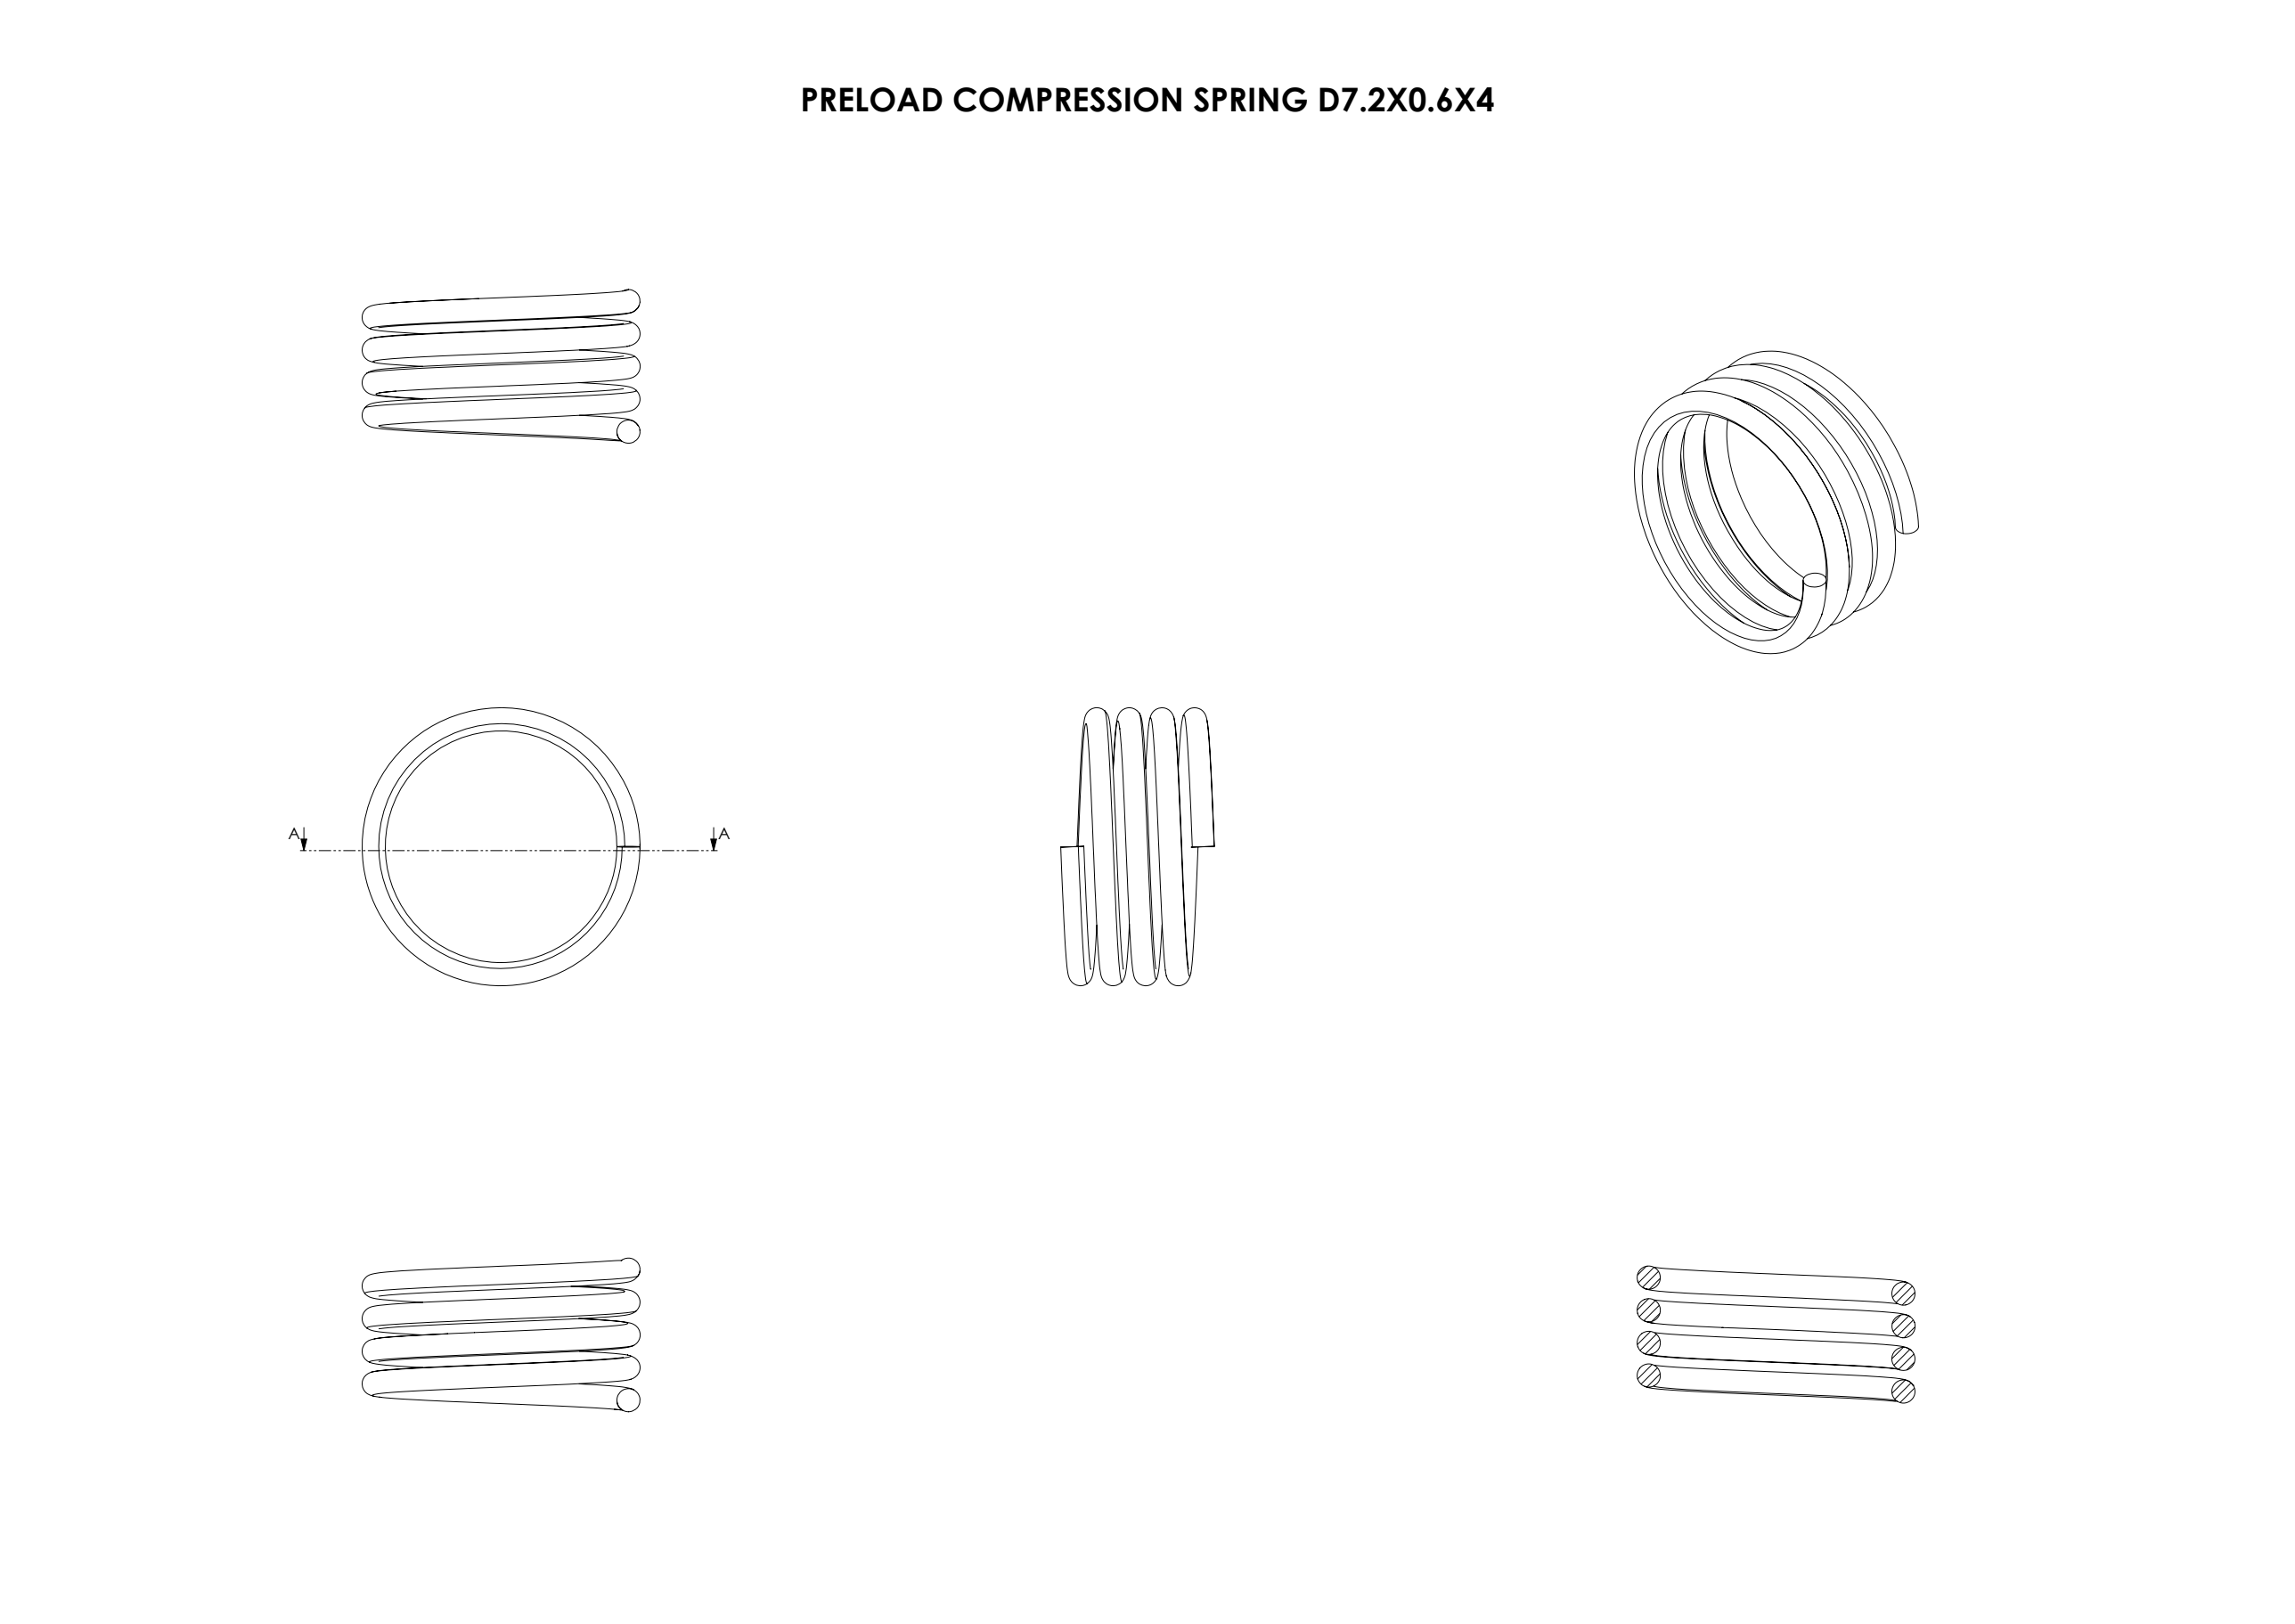
ISO-10303-21;
HEADER;
/* Generated by software containing ST-Developer
 * from STEP Tools, Inc. (www.steptools.com) 
 */

FILE_DESCRIPTION(
/* description */ (''),
/* implementation_level */ '2;1');

FILE_NAME(
/* name */ 
'10_Preload_Compression_Spring_D7.2x0.6x4.step',
/* time_stamp */ '2026-10-20T10:06:23-07:00',
/* author */ (''),
/* organization */ (''),
/* preprocessor_version */ 'ST-DEVELOPER v20.2',
/* originating_system */ 'Autodesk Translation Framework v15.15.0.0',
/* authorisation */ '');

FILE_SCHEMA (('AUTOMOTIVE_DESIGN { 1 0 10303 214 3 1 1 }'));
ENDSEC;

DATA;
#10=MECHANICAL_DESIGN_GEOMETRIC_PRESENTATION_REPRESENTATION('',(#471),#38611);
#443=SHAPE_REPRESENTATION_RELATIONSHIP('SRR','None',#38679,#457);
#457=ADVANCED_BREP_SHAPE_REPRESENTATION('',(#485),#38608);
#471=STYLED_ITEM('',(#38878),#485);
#485=MANIFOLD_SOLID_BREP('Spring',#16245);
#505=B_SPLINE_SURFACE_WITH_KNOTS('',3,3,((#31614,#31615,#31616,#31617,#31618,
#31619,#31620,#31621,#31622,#31623,#31624,#31625,#31626,#31627,#31628,#31629,
#31630,#31631,#31632,#31633,#31634,#31635,#31636,#31637,#31638,#31639,#31640,
#31641,#31642,#31643,#31644,#31645,#31646,#31647,#31648,#31649,#31650,#31651,
#31652,#31653,#31654,#31655,#31656,#31657,#31658,#31659,#31660,#31661,#31662,
#31663,#31664,#31665,#31666,#31667),(#31668,#31669,#31670,#31671,#31672,
#31673,#31674,#31675,#31676,#31677,#31678,#31679,#31680,#31681,#31682,#31683,
#31684,#31685,#31686,#31687,#31688,#31689,#31690,#31691,#31692,#31693,#31694,
#31695,#31696,#31697,#31698,#31699,#31700,#31701,#31702,#31703,#31704,#31705,
#31706,#31707,#31708,#31709,#31710,#31711,#31712,#31713,#31714,#31715,#31716,
#31717,#31718,#31719,#31720,#31721),(#31722,#31723,#31724,#31725,#31726,
#31727,#31728,#31729,#31730,#31731,#31732,#31733,#31734,#31735,#31736,#31737,
#31738,#31739,#31740,#31741,#31742,#31743,#31744,#31745,#31746,#31747,#31748,
#31749,#31750,#31751,#31752,#31753,#31754,#31755,#31756,#31757,#31758,#31759,
#31760,#31761,#31762,#31763,#31764,#31765,#31766,#31767,#31768,#31769,#31770,
#31771,#31772,#31773,#31774,#31775),(#31776,#31777,#31778,#31779,#31780,
#31781,#31782,#31783,#31784,#31785,#31786,#31787,#31788,#31789,#31790,#31791,
#31792,#31793,#31794,#31795,#31796,#31797,#31798,#31799,#31800,#31801,#31802,
#31803,#31804,#31805,#31806,#31807,#31808,#31809,#31810,#31811,#31812,#31813,
#31814,#31815,#31816,#31817,#31818,#31819,#31820,#31821,#31822,#31823,#31824,
#31825,#31826,#31827,#31828,#31829),(#31830,#31831,#31832,#31833,#31834,
#31835,#31836,#31837,#31838,#31839,#31840,#31841,#31842,#31843,#31844,#31845,
#31846,#31847,#31848,#31849,#31850,#31851,#31852,#31853,#31854,#31855,#31856,
#31857,#31858,#31859,#31860,#31861,#31862,#31863,#31864,#31865,#31866,#31867,
#31868,#31869,#31870,#31871,#31872,#31873,#31874,#31875,#31876,#31877,#31878,
#31879,#31880,#31881,#31882,#31883),(#31884,#31885,#31886,#31887,#31888,
#31889,#31890,#31891,#31892,#31893,#31894,#31895,#31896,#31897,#31898,#31899,
#31900,#31901,#31902,#31903,#31904,#31905,#31906,#31907,#31908,#31909,#31910,
#31911,#31912,#31913,#31914,#31915,#31916,#31917,#31918,#31919,#31920,#31921,
#31922,#31923,#31924,#31925,#31926,#31927,#31928,#31929,#31930,#31931,#31932,
#31933,#31934,#31935,#31936,#31937),(#31938,#31939,#31940,#31941,#31942,
#31943,#31944,#31945,#31946,#31947,#31948,#31949,#31950,#31951,#31952,#31953,
#31954,#31955,#31956,#31957,#31958,#31959,#31960,#31961,#31962,#31963,#31964,
#31965,#31966,#31967,#31968,#31969,#31970,#31971,#31972,#31973,#31974,#31975,
#31976,#31977,#31978,#31979,#31980,#31981,#31982,#31983,#31984,#31985,#31986,
#31987,#31988,#31989,#31990,#31991),(#31992,#31993,#31994,#31995,#31996,
#31997,#31998,#31999,#32000,#32001,#32002,#32003,#32004,#32005,#32006,#32007,
#32008,#32009,#32010,#32011,#32012,#32013,#32014,#32015,#32016,#32017,#32018,
#32019,#32020,#32021,#32022,#32023,#32024,#32025,#32026,#32027,#32028,#32029,
#32030,#32031,#32032,#32033,#32034,#32035,#32036,#32037,#32038,#32039,#32040,
#32041,#32042,#32043,#32044,#32045),(#32046,#32047,#32048,#32049,#32050,
#32051,#32052,#32053,#32054,#32055,#32056,#32057,#32058,#32059,#32060,#32061,
#32062,#32063,#32064,#32065,#32066,#32067,#32068,#32069,#32070,#32071,#32072,
#32073,#32074,#32075,#32076,#32077,#32078,#32079,#32080,#32081,#32082,#32083,
#32084,#32085,#32086,#32087,#32088,#32089,#32090,#32091,#32092,#32093,#32094,
#32095,#32096,#32097,#32098,#32099),(#32100,#32101,#32102,#32103,#32104,
#32105,#32106,#32107,#32108,#32109,#32110,#32111,#32112,#32113,#32114,#32115,
#32116,#32117,#32118,#32119,#32120,#32121,#32122,#32123,#32124,#32125,#32126,
#32127,#32128,#32129,#32130,#32131,#32132,#32133,#32134,#32135,#32136,#32137,
#32138,#32139,#32140,#32141,#32142,#32143,#32144,#32145,#32146,#32147,#32148,
#32149,#32150,#32151,#32152,#32153),(#32154,#32155,#32156,#32157,#32158,
#32159,#32160,#32161,#32162,#32163,#32164,#32165,#32166,#32167,#32168,#32169,
#32170,#32171,#32172,#32173,#32174,#32175,#32176,#32177,#32178,#32179,#32180,
#32181,#32182,#32183,#32184,#32185,#32186,#32187,#32188,#32189,#32190,#32191,
#32192,#32193,#32194,#32195,#32196,#32197,#32198,#32199,#32200,#32201,#32202,
#32203,#32204,#32205,#32206,#32207)),.UNSPECIFIED.,.T.,.F.,.F.,(4,1,1,1,
1,1,1,1,4),(4,1,1,1,1,1,1,1,1,1,1,1,1,1,1,1,1,1,1,1,1,1,1,1,1,1,1,1,1,1,
1,1,1,1,1,1,1,1,1,1,1,1,1,1,1,1,1,1,1,1,1,4),(-3.14159265358979,-2.46839422782055,
-2.24399475256414,-1.34639685153848,-0.448798950512828,0.448798950512828,
1.34639685153848,2.24399475256414,3.14159265358979),(0.,0.0178571428571429,
0.0357142857142857,0.0535714285714286,0.0714285714285714,0.0892857142857143,
0.107142857142857,0.125,0.133928571428571,0.138392857142857,0.142857142857143,
0.166666666666667,0.19047619047619,0.214285714285714,0.232142857142857,
0.25,0.267857142857143,0.285714285714286,0.303571428571429,0.321428571428571,
0.339285714285714,0.357142857142857,0.375,0.392857142857143,0.428571428571429,
0.464285714285714,0.5,0.535714285714286,0.553571428571429,0.571428571428571,
0.589285714285714,0.607142857142857,0.625,0.642857142857143,0.660714285714286,
0.678571428571428,0.696428571428571,0.714285714285714,0.738095238095238,
0.761904761904762,0.785714285714286,0.809523809523809,0.833333333333333,
0.857142857142857,0.875,0.892857142857143,0.910714285714286,0.928571428571429,
0.946428571428571,0.964285714285714,0.982142857142857,1.),.UNSPECIFIED.);
#728=B_SPLINE_CURVE_WITH_KNOTS('',3,(#32211,#32212,#32213,#32214,#32215,
#32216,#32217,#32218,#32219,#32220,#32221,#32222,#32223,#32224,#32225,#32226,
#32227,#32228,#32229,#32230,#32231,#32232,#32233,#32234,#32235,#32236,#32237,
#32238,#32239,#32240,#32241,#32242,#32243,#32244,#32245,#32246,#32247,#32248,
#32249,#32250,#32251,#32252,#32253,#32254,#32255,#32256,#32257,#32258,#32259,
#32260,#32261,#32262,#32263,#32264),.UNSPECIFIED.,.F.,.F.,(4,1,1,1,1,1,
1,1,1,1,1,1,1,1,1,1,1,1,1,1,1,1,1,1,1,1,1,1,1,1,1,1,1,1,1,1,1,1,1,1,1,1,
1,1,1,1,1,1,1,1,1,4),(0.,0.0178571428571429,0.0357142857142857,0.0535714285714286,
0.0714285714285714,0.0892857142857143,0.107142857142857,0.125,0.133928571428571,
0.138392857142857,0.142857142857143,0.166666666666667,0.19047619047619,
0.214285714285714,0.232142857142857,0.25,0.267857142857143,0.285714285714286,
0.303571428571429,0.321428571428571,0.339285714285714,0.357142857142857,
0.375,0.392857142857143,0.428571428571429,0.464285714285714,0.5,0.535714285714286,
0.553571428571429,0.571428571428571,0.589285714285714,0.607142857142857,
0.625,0.642857142857143,0.660714285714286,0.678571428571428,0.696428571428571,
0.714285714285714,0.738095238095238,0.761904761904762,0.785714285714286,
0.809523809523809,0.833333333333333,0.857142857142857,0.875,0.892857142857143,
0.910714285714286,0.928571428571429,0.946428571428571,0.964285714285714,
0.982142857142857,1.),.UNSPECIFIED.);
#1516=CIRCLE('',#17328,0.03);
#1517=CIRCLE('',#17329,0.03);
#2388=FACE_OUTER_BOUND('',#3348,.T.);
#2389=FACE_OUTER_BOUND('',#3349,.T.);
#2390=FACE_OUTER_BOUND('',#3350,.T.);
#3348=EDGE_LOOP('',(#13117,#13118,#13119,#13120));
#3349=EDGE_LOOP('',(#13121));
#3350=EDGE_LOOP('',(#13122));
#7074=VERTEX_POINT('',#32208);
#7075=VERTEX_POINT('',#32210);
#9174=EDGE_CURVE('',#7074,#7074,#1516,.T.);
#9175=EDGE_CURVE('',#7074,#7075,#728,.T.);
#9176=EDGE_CURVE('',#7075,#7075,#1517,.T.);
#13117=ORIENTED_EDGE('',*,*,#9174,.T.);
#13118=ORIENTED_EDGE('',*,*,#9175,.T.);
#13119=ORIENTED_EDGE('',*,*,#9176,.F.);
#13120=ORIENTED_EDGE('',*,*,#9175,.F.);
#13121=ORIENTED_EDGE('',*,*,#9176,.T.);
#13122=ORIENTED_EDGE('',*,*,#9174,.F.);
#15156=PLANE('',#17330);
#15157=PLANE('',#17331);
#15931=ADVANCED_FACE('',(#2388),#505,.T.);
#15932=ADVANCED_FACE('',(#2389),#15156,.T.);
#15933=ADVANCED_FACE('',(#2390),#15157,.F.);
#16245=CLOSED_SHELL('',(#15931,#15932,#15933));
#17327=AXIS2_PLACEMENT_3D('',#31613,#20517,#20518);
#17328=AXIS2_PLACEMENT_3D('',#32209,#20519,#20520);
#17329=AXIS2_PLACEMENT_3D('',#32265,#20521,#20522);
#17330=AXIS2_PLACEMENT_3D('',#32266,#20523,#20524);
#17331=AXIS2_PLACEMENT_3D('',#32267,#20525,#20526);
#20517=DIRECTION('axis',(0.,0.,1.));
#20518=DIRECTION('refdir',(1.,0.,0.));
#20519=DIRECTION('center_axis',(-0.00361045998153645,0.999206964682131,
0.0396535787722272));
#20520=DIRECTION('ref_axis',(0.000143280351062803,-0.0396533199138007,0.999213487544356));
#20521=DIRECTION('center_axis',(0.00361045998921086,0.999206964681458,0.0396535787884862));
#20522=DIRECTION('ref_axis',(-0.853800279921239,-0.017563245976609,0.520304347855348));
#20523=DIRECTION('center_axis',(0.00361045998921086,0.999206964681458,0.0396535787884862));
#20524=DIRECTION('ref_axis',(-0.853800279921239,-0.017563245976609,0.520304347855348));
#20525=DIRECTION('center_axis',(-0.00361045998153645,0.999206964682131,
0.0396535787722272));
#20526=DIRECTION('ref_axis',(0.000143280351062803,-0.0396533199138007,0.999213487544356));
#31613=CARTESIAN_POINT('',(0.,0.,0.));
#31614=CARTESIAN_POINT('Ctrl Pts',(0.329995701589468,0.00118959959741402,
0.00102359537366932));
#31615=CARTESIAN_POINT('Ctrl Pts',(0.329812358348379,0.0519304593106012,
0.00303724894968045));
#31616=CARTESIAN_POINT('Ctrl Pts',(0.307603150250096,0.14856309907024,0.007063921474547));
#31617=CARTESIAN_POINT('Ctrl Pts',(0.212522007054295,0.2688270154723,0.0131144005095069));
#31618=CARTESIAN_POINT('Ctrl Pts',(0.0751961041762406,0.33443845631537,
0.0191752186885983));
#31619=CARTESIAN_POINT('Ctrl Pts',(-0.0776142387319525,0.334810528053721,
0.025245738062024));
#31620=CARTESIAN_POINT('Ctrl Pts',(-0.215432226705683,0.268236493442132,
0.0313264548832147));
#31621=CARTESIAN_POINT('Ctrl Pts',(-0.311063582237146,0.148538498980413,
0.0374170400486292));
#31622=CARTESIAN_POINT('Ctrl Pts',(-0.339534702539374,0.0237758430999062,
0.0425008539245673));
#31623=CARTESIAN_POINT('Ctrl Pts',(-0.329617478537296,-0.0636510452603832,
0.0460638560210726));
#31624=CARTESIAN_POINT('Ctrl Pts',(-0.315752180564557,-0.111758567679568,
0.0481010960909614));
#31625=CARTESIAN_POINT('Ctrl Pts',(-0.280687728436729,-0.19663499457563,
0.0518375549362775));
#31626=CARTESIAN_POINT('Ctrl Pts',(-0.176953832876605,-0.308707864139412,
0.0577895429568186));
#31627=CARTESIAN_POINT('Ctrl Pts',(0.0277912542949835,-0.355359243876355,
0.0659698006169508));
#31628=CARTESIAN_POINT('Ctrl Pts',(0.207256209567046,-0.285022432777545,
0.073484386523706));
#31629=CARTESIAN_POINT('Ctrl Pts',(0.31450859302708,-0.150158997366471,
0.0803284879538114));
#31630=CARTESIAN_POINT('Ctrl Pts',(0.349186611535958,0.00111014849211965,
0.0864979120385476));
#31631=CARTESIAN_POINT('Ctrl Pts',(0.314520756767304,0.152731777144028,
0.0926770234710082));
#31632=CARTESIAN_POINT('Ctrl Pts',(0.217500483746742,0.274539465175591,
0.098865768103921));
#31633=CARTESIAN_POINT('Ctrl Pts',(0.0769551264679099,0.342186713109751,
0.105064101576398));
#31634=CARTESIAN_POINT('Ctrl Pts',(-0.0793009475509065,0.342263708237282,
0.111271969453101));
#31635=CARTESIAN_POINT('Ctrl Pts',(-0.220172034550062,0.274381760656883,
0.117489309777858));
#31636=CARTESIAN_POINT('Ctrl Pts',(-0.318128621603507,0.151819046241454,
0.123716067105663));
#31637=CARTESIAN_POINT('Ctrl Pts',(-0.352617648223723,-0.000927697002303161,
0.129952164368648));
#31638=CARTESIAN_POINT('Ctrl Pts',(-0.307197248189229,-0.205991895653557,
0.138279361997572));
#31639=CARTESIAN_POINT('Ctrl Pts',(-0.0867093646975666,-0.382606488631909,
0.148711360096893));
#31640=CARTESIAN_POINT('Ctrl Pts',(0.246157896760925,-0.307226237821677,
0.16126605881999));
#31641=CARTESIAN_POINT('Ctrl Pts',(0.394548713993526,0.00121213976701099,
0.173856329664019));
#31642=CARTESIAN_POINT('Ctrl Pts',(0.270683494680064,0.25779707362797,0.184377360469391));
#31643=CARTESIAN_POINT('Ctrl Pts',(0.0784480660104459,0.348945360245205,
0.192811248605432));
#31644=CARTESIAN_POINT('Ctrl Pts',(-0.0805931042682236,0.349358375490888,
0.199145126960344));
#31645=CARTESIAN_POINT('Ctrl Pts',(-0.224524686851408,0.279914574363962,
0.205487348255157));
#31646=CARTESIAN_POINT('Ctrl Pts',(-0.324178791380424,0.155094279198964,
0.211837815149481));
#31647=CARTESIAN_POINT('Ctrl Pts',(-0.359765231562575,-0.000950160030172512,
0.218196411362682));
#31648=CARTESIAN_POINT('Ctrl Pts',(-0.324199918380757,-0.157162565812712,
0.22456305908972));
#31649=CARTESIAN_POINT('Ctrl Pts',(-0.224151419632265,-0.282543079616346,
0.230937631934188));
#31650=CARTESIAN_POINT('Ctrl Pts',(-0.0794762745603369,-0.352337612459348,
0.237319995378052));
#31651=CARTESIAN_POINT('Ctrl Pts',(0.0812906306420514,-0.352242766117238,
0.243710053380832));
#31652=CARTESIAN_POINT('Ctrl Pts',(0.242583044989387,-0.274824345329341,
0.250818566710242));
#31653=CARTESIAN_POINT('Ctrl Pts',(0.355857692111688,-0.108936398125315,
0.258648506513342));
#31654=CARTESIAN_POINT('Ctrl Pts',(0.35601905515454,0.110643209305051,0.267203260973594));
#31655=CARTESIAN_POINT('Ctrl Pts',(0.232065828412221,0.292295611594562,
0.275770669585301));
#31656=CARTESIAN_POINT('Ctrl Pts',(0.0272435837717024,0.37290401539681,
0.284350408116761));
#31657=CARTESIAN_POINT('Ctrl Pts',(-0.187879927304316,0.323810447294939,
0.292942183858905));
#31658=CARTESIAN_POINT('Ctrl Pts',(-0.325407735789747,0.17542191209667,
0.300828814614272));
#31659=CARTESIAN_POINT('Ctrl Pts',(-0.365431318619722,-0.00075089577638709,
0.308006589851792));
#31660=CARTESIAN_POINT('Ctrl Pts',(-0.329362034481868,-0.159416832712907,
0.314473213303831));
#31661=CARTESIAN_POINT('Ctrl Pts',(-0.227729428899003,-0.286678573326201,
0.320945361203317));
#31662=CARTESIAN_POINT('Ctrl Pts',(-0.0809152203341978,-0.357609127112455,
0.327424927538347));
#31663=CARTESIAN_POINT('Ctrl Pts',(0.0823028008577847,-0.357312684079966,
0.333907107762849));
#31664=CARTESIAN_POINT('Ctrl Pts',(0.229369976399687,-0.286999416296364,
0.340400245782608));
#31665=CARTESIAN_POINT('Ctrl Pts',(0.331477217034357,-0.158117971828307,
0.346888605564388));
#31666=CARTESIAN_POINT('Ctrl Pts',(0.355417803964002,-0.0537733405890617,
0.351235961881927));
#31667=CARTESIAN_POINT('Ctrl Pts',(0.355614008397637,0.000526897379297947,
0.35339086956434));
#31668=CARTESIAN_POINT('Ctrl Pts',(0.323263761278146,0.0011652749059825,
0.00102359537366932));
#31669=CARTESIAN_POINT('Ctrl Pts',(0.32308388504024,0.0509466298067978,
0.00299917095282439));
#31670=CARTESIAN_POINT('Ctrl Pts',(0.301325186385381,0.145526233085643,
0.0069406494446651));
#31671=CARTESIAN_POINT('Ctrl Pts',(0.208169819552591,0.263398218702504,
0.0128703570176973));
#31672=CARTESIAN_POINT('Ctrl Pts',(0.0736352659440483,0.327653486273809,
0.0188072832941143));
#31673=CARTESIAN_POINT('Ctrl Pts',(-0.0760885903995774,0.328030617131512,
0.0247556929444235));
#31674=CARTESIAN_POINT('Ctrl Pts',(-0.211125322474165,0.262793911768754,
0.0307136354236982));
#31675=CARTESIAN_POINT('Ctrl Pts',(-0.30483335192296,0.145508174571446,
0.0366818386650944));
#31676=CARTESIAN_POINT('Ctrl Pts',(-0.332736604267165,0.0232418188678019,
0.0416639718287818));
#31677=CARTESIAN_POINT('Ctrl Pts',(-0.3230187894293,-0.0624385261228433,
0.0451558754794785));
#31678=CARTESIAN_POINT('Ctrl Pts',(-0.309430912508696,-0.10958390059491,
0.0471523807534524));
#31679=CARTESIAN_POINT('Ctrl Pts',(-0.275067160512545,-0.192765131089754,
0.0508142216208795));
#31680=CARTESIAN_POINT('Ctrl Pts',(-0.173384898218217,-0.30262257252764,
0.0566489427637022));
#31681=CARTESIAN_POINT('Ctrl Pts',(0.0273145804812777,-0.348359213768784,
0.0646675914287231));
#31682=CARTESIAN_POINT('Ctrl Pts',(0.203266956937511,-0.279400513558744,
0.0720353597363947));
#31683=CARTESIAN_POINT('Ctrl Pts',(0.308436007640621,-0.147165797018185,
0.0787463017504538));
#31684=CARTESIAN_POINT('Ctrl Pts',(0.342442191511722,0.00117726716011259,
0.0847965020332884));
#31685=CARTESIAN_POINT('Ctrl Pts',(0.308448294174871,0.149886349764988,
0.0908569625697496));
#31686=CARTESIAN_POINT('Ctrl Pts',(0.213279665334743,0.26936826303577,0.0969276519284122));
#31687=CARTESIAN_POINT('Ctrl Pts',(0.0754008583417468,0.335738815799705,
0.103008616752156));
#31688=CARTESIAN_POINT('Ctrl Pts',(-0.0779153548107563,0.335814356976075,
0.109099752247069));
#31689=CARTESIAN_POINT('Ctrl Pts',(-0.216159240659499,0.269204901675787,
0.115201143937647));
#31690=CARTESIAN_POINT('Ctrl Pts',(-0.312302840736801,0.148912374598733,
0.121312645115956));
#31691=CARTESIAN_POINT('Ctrl Pts',(-0.346163600796807,-0.00102923428505851,
0.127434365100191));
#31692=CARTESIAN_POINT('Ctrl Pts',(-0.301573902044757,-0.202360103152527,
0.135610016965582));
#31693=CARTESIAN_POINT('Ctrl Pts',(-0.0850566432589637,-0.375824958530099,
0.145855089726598));
#31694=CARTESIAN_POINT('Ctrl Pts',(0.241962386947492,-0.301799047216122,
0.158189044407346));
#31695=CARTESIAN_POINT('Ctrl Pts',(0.387828938012594,0.00131775672787745,
0.170562769165271));
#31696=CARTESIAN_POINT('Ctrl Pts',(0.266068485484251,0.253601605330286,
0.180906998748366));
#31697=CARTESIAN_POINT('Ctrl Pts',(0.0770061287527791,0.343252947438917,
0.189201773157529));
#31698=CARTESIAN_POINT('Ctrl Pts',(-0.0794446669689747,0.343662665319532,
0.195432501073281));
#31699=CARTESIAN_POINT('Ctrl Pts',(-0.221066126232674,0.275338906399848,
0.201672855000828));
#31700=CARTESIAN_POINT('Ctrl Pts',(-0.319144627584919,0.152499087945336,
0.207922683407449));
#31701=CARTESIAN_POINT('Ctrl Pts',(-0.354179786673318,-0.00110753927353714,
0.214182002780984));
#31702=CARTESIAN_POINT('Ctrl Pts',(-0.319166531156333,-0.154917399863823,
0.220450660338253));
#31703=CARTESIAN_POINT('Ctrl Pts',(-0.220637111918073,-0.278401206258936,
0.226728661851426));
#31704=CARTESIAN_POINT('Ctrl Pts',(-0.0781215508622231,-0.347159715044341,
0.233015834255785));
#31705=CARTESIAN_POINT('Ctrl Pts',(0.080287554663607,-0.347070588075095,
0.239312154857787));
#31706=CARTESIAN_POINT('Ctrl Pts',(0.239257652256424,-0.270773321076525,
0.246318192490788));
#31707=CARTESIAN_POINT('Ctrl Pts',(0.35093898589305,-0.107236396197418,
0.254037368004576));
#31708=CARTESIAN_POINT('Ctrl Pts',(0.351111227440523,0.10931883915664,0.262474266548859));
#31709=CARTESIAN_POINT('Ctrl Pts',(0.228833468081611,0.288535277900801,
0.270926380939377));
#31710=CARTESIAN_POINT('Ctrl Pts',(0.0266925824577831,0.368103565438035,
0.279393970650793));
#31711=CARTESIAN_POINT('Ctrl Pts',(-0.185696236216694,0.319645295407652,
0.287876328764416));
#31712=CARTESIAN_POINT('Ctrl Pts',(-0.321535144076036,0.173101071392216,
0.295665258245558));
#31713=CARTESIAN_POINT('Ctrl Pts',(-0.361082579337844,-0.000956223706756918,
0.302756882611919));
#31714=CARTESIAN_POINT('Ctrl Pts',(-0.32544517604417,-0.157762357732159,
0.309147439370426));
#31715=CARTESIAN_POINT('Ctrl Pts',(-0.224978122399143,-0.283567336452126,
0.315545488109766));
#31716=CARTESIAN_POINT('Ctrl Pts',(-0.0798082459991771,-0.353718739900048,
0.32195248587614));
#31717=CARTESIAN_POINT('Ctrl Pts',(0.0816387315204158,-0.353420513894944,
0.328364404520402));
#31718=CARTESIAN_POINT('Ctrl Pts',(0.227155226998822,-0.283871579779252,
0.334788486194004));
#31719=CARTESIAN_POINT('Ctrl Pts',(0.328215224283278,-0.156290050231924,
0.341210885809922));
#31720=CARTESIAN_POINT('Ctrl Pts',(0.351915021246625,-0.0530322184023736,
0.345513041507324));
#31721=CARTESIAN_POINT('Ctrl Pts',(0.35210941700762,0.000767463320028059,
0.347648084589869));
#31722=CARTESIAN_POINT('Ctrl Pts',(0.3143497770318,0.00100791399453752,
0.00417722082587345));
#31723=CARTESIAN_POINT('Ctrl Pts',(0.314174444955958,0.0495316567334979,
0.006102888002978));
#31724=CARTESIAN_POINT('Ctrl Pts',(0.293026748720441,0.141376025106581,
0.00993052643649342));
#31725=CARTESIAN_POINT('Ctrl Pts',(0.202454346374076,0.256059066455207,
0.0156981800761764));
#31726=CARTESIAN_POINT('Ctrl Pts',(0.0716524230376314,0.318486601600921,
0.0214690413557031));
#31727=CARTESIAN_POINT('Ctrl Pts',(-0.0739017686534995,0.31887794641969,
0.0272520660610699));
#31728=CARTESIAN_POINT('Ctrl Pts',(-0.205150715552183,0.255448411785207,
0.0330425408443067));
#31729=CARTESIAN_POINT('Ctrl Pts',(-0.296232579005206,0.141460288765413,
0.0388433659915622));
#31730=CARTESIAN_POINT('Ctrl Pts',(-0.323344939862462,0.0226317046800233,
0.0436848833441879));
#31731=CARTESIAN_POINT('Ctrl Pts',(-0.313899608979832,-0.060631936346867,
0.0470782603736746));
#31732=CARTESIAN_POINT('Ctrl Pts',(-0.300693617065818,-0.106451761520664,
0.0490185943697462));
#31733=CARTESIAN_POINT('Ctrl Pts',(-0.267296784696181,-0.187291053982876,
0.0525773313312681));
#31734=CARTESIAN_POINT('Ctrl Pts',(-0.168501916293235,-0.294031184492012,
0.0582458003866922));
#31735=CARTESIAN_POINT('Ctrl Pts',(0.0265217080425736,-0.338468900053865,
0.066037693415352));
#31736=CARTESIAN_POINT('Ctrl Pts',(0.197480954357712,-0.271470453852949,
0.0731959148965402));
#31737=CARTESIAN_POINT('Ctrl Pts',(0.299662458425762,-0.1429841872325,0.0797163664559953));
#31738=CARTESIAN_POINT('Ctrl Pts',(0.332707595799803,0.00114716748899207,
0.0855946560055489));
#31739=CARTESIAN_POINT('Ctrl Pts',(0.299673735812974,0.145633690283821,
0.0914829317886208));
#31740=CARTESIAN_POINT('Ctrl Pts',(0.207208825230489,0.261728500340961,
0.097381253187885));
#31741=CARTESIAN_POINT('Ctrl Pts',(0.0732372745429245,0.326212791260178,
0.103289636985298));
#31742=CARTESIAN_POINT('Ctrl Pts',(-0.0757368242826929,0.326290610457155,
0.109208166354362));
#31743=CARTESIAN_POINT('Ctrl Pts',(-0.210069264644612,0.261561190313174,
0.115136835302027));
#31744=CARTESIAN_POINT('Ctrl Pts',(-0.303501461520976,0.144667206221031,
0.121075735274062));
#31745=CARTESIAN_POINT('Ctrl Pts',(-0.33640552849753,-0.00105114360770151,
0.127024838842762));
#31746=CARTESIAN_POINT('Ctrl Pts',(-0.293071888244684,-0.196725338364434,
0.134970722603791));
#31747=CARTESIAN_POINT('Ctrl Pts',(-0.0826205547868334,-0.365337759369106,
0.144928659779304));
#31748=CARTESIAN_POINT('Ctrl Pts',(0.235308544687022,-0.293385579417626,
0.156919602308117));
#31749=CARTESIAN_POINT('Ctrl Pts',(0.377167918354085,0.00136502922110808,
0.168951937351355));
#31750=CARTESIAN_POINT('Ctrl Pts',(0.258748526764981,0.246762198818122,
0.179013431660086));
#31751=CARTESIAN_POINT('Ctrl Pts',(0.0748100498926877,0.333987556781711,
0.187083384029882));
#31752=CARTESIAN_POINT('Ctrl Pts',(-0.0774247661752075,0.334388365324906,
0.193146211385528));
#31753=CARTESIAN_POINT('Ctrl Pts',(-0.215253722800486,0.267896699637554,
0.199219373691256));
#31754=CARTESIAN_POINT('Ctrl Pts',(-0.310723951021264,0.148327693877378,
0.205302893635305));
#31755=CARTESIAN_POINT('Ctrl Pts',(-0.344835425098166,-0.0012174970511246,
0.211396712812984));
#31756=CARTESIAN_POINT('Ctrl Pts',(-0.310743621977528,-0.150990654519629,
0.217500860527999));
#31757=CARTESIAN_POINT('Ctrl Pts',(-0.214783997648992,-0.271259017547068,
0.22361526923801));
#31758=CARTESIAN_POINT('Ctrl Pts',(-0.0759539911741114,-0.338242375219202,
0.229739944634851));
#31759=CARTESIAN_POINT('Ctrl Pts',(0.0783932441541543,-0.338159167803166,
0.235874832502872));
#31760=CARTESIAN_POINT('Ctrl Pts',(0.233321229982812,-0.263805853805254,
0.24270269913196));
#31761=CARTESIAN_POINT('Ctrl Pts',(0.342201575184436,-0.104386212514232,
0.250227870691107));
#31762=CARTESIAN_POINT('Ctrl Pts',(0.342377862772396,0.10678419186207,0.258455044914927));
#31763=CARTESIAN_POINT('Ctrl Pts',(0.223106451745026,0.281615630068196,
0.266700149646066));
#31764=CARTESIAN_POINT('Ctrl Pts',(0.0258611457879684,0.359265028954348,
0.274962893164122));
#31765=CARTESIAN_POINT('Ctrl Pts',(-0.181471173906832,0.311975315176289,
0.283243312867527));
#31766=CARTESIAN_POINT('Ctrl Pts',(-0.314129400185778,0.168869863676765,
0.290849825356883));
#31767=CARTESIAN_POINT('Ctrl Pts',(-0.352767893347067,-0.0011524177295687,
0.297777211902988));
#31768=CARTESIAN_POINT('Ctrl Pts',(-0.317947143101735,-0.154378046283838,
0.304021816820379));
#31769=CARTESIAN_POINT('Ctrl Pts',(-0.219751851958905,-0.2773449048768,
0.310275672881377));
#31770=CARTESIAN_POINT('Ctrl Pts',(-0.0778177620146979,-0.345946144519262,
0.316539857977124));
#31771=CARTESIAN_POINT('Ctrl Pts',(0.0800916001784434,-0.345646777099896,
0.322811784793249));
#31772=CARTESIAN_POINT('Ctrl Pts',(0.222457203835381,-0.277635516145105,
0.329095893848701));
#31773=CARTESIAN_POINT('Ctrl Pts',(0.321375732078151,-0.152720989873198,
0.335383674313783));
#31774=CARTESIAN_POINT('Ctrl Pts',(0.344583361544119,-0.0517156352897094,
0.339592387805982));
#31775=CARTESIAN_POINT('Ctrl Pts',(0.344773950821541,0.00103058928075043,
0.341685624388322));
#31776=CARTESIAN_POINT('Ctrl Pts',(0.301487309249758,0.000456552091686937,
0.0168995335103255));
#31777=CARTESIAN_POINT('Ctrl Pts',(0.301318644157645,0.0471351846205436,
0.0187519773957139));
#31778=CARTESIAN_POINT('Ctrl Pts',(0.2810381206102,0.135021677602031,0.0224153073649692));
#31779=CARTESIAN_POINT('Ctrl Pts',(0.194239037473508,0.245007882920672,
0.027945676794797));
#31780=CARTESIAN_POINT('Ctrl Pts',(0.0689981063776347,0.304715578239823,
0.0334693902717626));
#31781=CARTESIAN_POINT('Ctrl Pts',(-0.0702900555082151,0.305109671029292,
0.0390042903358426));
#31782=CARTESIAN_POINT('Ctrl Pts',(-0.195787398577806,0.244427515329891,
0.044540988571053));
#31783=CARTESIAN_POINT('Ctrl Pts',(-0.282824724120957,0.135496598851049,
0.0500848449251036));
#31784=CARTESIAN_POINT('Ctrl Pts',(-0.308711795376669,0.0219958303263355,
0.0547090024061654));
#31785=CARTESIAN_POINT('Ctrl Pts',(-0.29969420448995,-0.0574925396160197,
0.0579486413010252));
#31786=CARTESIAN_POINT('Ctrl Pts',(-0.287089894521034,-0.101224391094012,
0.0598005555602701));
#31787=CARTESIAN_POINT('Ctrl Pts',(-0.255219231588607,-0.178368997813358,
0.0631966456490891));
#31788=CARTESIAN_POINT('Ctrl Pts',(-0.160958434699617,-0.280185707839856,
0.0686045510379543));
#31789=CARTESIAN_POINT('Ctrl Pts',(0.0249425970611792,-0.322526026192247,
0.0760318037970623));
#31790=CARTESIAN_POINT('Ctrl Pts',(0.187788206134099,-0.258686428390149,
0.0828508087168802));
#31791=CARTESIAN_POINT('Ctrl Pts',(0.285061784518795,-0.136361708668944,
0.0890584674717641));
#31792=CARTESIAN_POINT('Ctrl Pts',(0.316497406441131,0.000792437315105745,
0.0946521949347518));
#31793=CARTESIAN_POINT('Ctrl Pts',(0.28507324950853,0.138219078024721,0.100252882809767));
#31794=CARTESIAN_POINT('Ctrl Pts',(0.197156599915038,0.248588740509545,
0.105860686505017));
#31795=CARTESIAN_POINT('Ctrl Pts',(0.0698367774737854,0.309867367627101,
0.111475746073964));
#31796=CARTESIAN_POINT('Ctrl Pts',(-0.0716830353582476,0.309933053031314,
0.117098178038573));
#31797=CARTESIAN_POINT('Ctrl Pts',(-0.199244451681163,0.248462891041503,
0.122728160853189));
#31798=CARTESIAN_POINT('Ctrl Pts',(-0.287930342488211,0.137494903576697,
0.128365781293317));
#31799=CARTESIAN_POINT('Ctrl Pts',(-0.319152161969064,-0.000783574171537168,
0.134011240827325));
#31800=CARTESIAN_POINT('Ctrl Pts',(-0.278035089510408,-0.18640701314818,
0.141548997600109));
#31801=CARTESIAN_POINT('Ctrl Pts',(-0.0784631926776667,-0.346266505185913,
0.150991489427036));
#31802=CARTESIAN_POINT('Ctrl Pts',(0.222836755126196,-0.278041772009318,
0.162355555259985));
#31803=CARTESIAN_POINT('Ctrl Pts',(0.357193668716545,0.00118449665979845,
0.17375385635394));
#31804=CARTESIAN_POINT('Ctrl Pts',(0.2450404452584,0.23355531905656,0.183281617763114));
#31805=CARTESIAN_POINT('Ctrl Pts',(0.0708989045308578,0.316131965777688,
0.190921795813857));
#31806=CARTESIAN_POINT('Ctrl Pts',(-0.0732099472936145,0.316509785082592,
0.196660991057498));
#31807=CARTESIAN_POINT('Ctrl Pts',(-0.203667301369978,0.253573050762465,
0.202409381813254));
#31808=CARTESIAN_POINT('Ctrl Pts',(-0.294022688408376,0.140408123958125,
0.208167033486851));
#31809=CARTESIAN_POINT('Ctrl Pts',(-0.326304383791802,-0.0011172174790417,
0.213934077022798));
#31810=CARTESIAN_POINT('Ctrl Pts',(-0.294042134324106,-0.142850802528825,
0.219710546097136));
#31811=CARTESIAN_POINT('Ctrl Pts',(-0.203236242617689,-0.256659822856353,
0.225496572304767));
#31812=CARTESIAN_POINT('Ctrl Pts',(-0.0718641880841615,-0.320045263581161,
0.231292227048866));
#31813=CARTESIAN_POINT('Ctrl Pts',(0.0741925396792679,-0.319966890116769,
0.237097594375026));
#31814=CARTESIAN_POINT('Ctrl Pts',(0.22080328921599,-0.249606394849742,
0.243558861586279));
#31815=CARTESIAN_POINT('Ctrl Pts',(0.323844093963753,-0.0987405175598124,
0.250680303919329));
#31816=CARTESIAN_POINT('Ctrl Pts',(0.32401507287333,0.101121051148882,0.258466870226901));
#31817=CARTESIAN_POINT('Ctrl Pts',(0.211121630360006,0.266610552139869,
0.266271226345274));
#31818=CARTESIAN_POINT('Ctrl Pts',(0.0243894520669469,0.340127943927118,
0.274093646786023));
#31819=CARTESIAN_POINT('Ctrl Pts',(-0.17192978881275,0.295356272268269,
0.28193413025846));
#31820=CARTESIAN_POINT('Ctrl Pts',(-0.297574955055663,0.159828459938204,
0.289137905336518));
#31821=CARTESIAN_POINT('Ctrl Pts',(-0.334179435288708,-0.0012318952504744,
0.295700328362607));
#31822=CARTESIAN_POINT('Ctrl Pts',(-0.301195173483201,-0.146417950178875,
0.301616739917366));
#31823=CARTESIAN_POINT('Ctrl Pts',(-0.208135055759231,-0.262944613995742,
0.307543700779419));
#31824=CARTESIAN_POINT('Ctrl Pts',(-0.0736043148012352,-0.328002669716722,
0.313480824491926));
#31825=CARTESIAN_POINT('Ctrl Pts',(0.0761330634504403,-0.327682926701522,
0.319429011228321));
#31826=CARTESIAN_POINT('Ctrl Pts',(0.211157784923481,-0.263255004979861,
0.325386838675828));
#31827=CARTESIAN_POINT('Ctrl Pts',(0.305008353090155,-0.144615638098925,
0.331356623228847));
#31828=CARTESIAN_POINT('Ctrl Pts',(0.327024456208159,-0.0489885211905165,
0.335341847701417));
#31829=CARTESIAN_POINT('Ctrl Pts',(0.327206044585182,0.00126667387289164,
0.337336227652134));
#31830=CARTESIAN_POINT('Ctrl Pts',(0.296534826482144,-0.000422773883966688,
0.0386062224122653));
#31831=CARTESIAN_POINT('Ctrl Pts',(0.296368800707151,0.0455254187392618,
0.0404296787531709));
#31832=CARTESIAN_POINT('Ctrl Pts',(0.276427070000758,0.131843682442671,
0.0440279011289847));
#31833=CARTESIAN_POINT('Ctrl Pts',(0.191202125564478,0.23985144495526,0.0494584217321202));
#31834=CARTESIAN_POINT('Ctrl Pts',(0.0684086392330356,0.298341986007322,
0.0548730358166816));
#31835=CARTESIAN_POINT('Ctrl Pts',(-0.0679772583367851,0.298725491344516,
0.0602928330160072));
#31836=CARTESIAN_POINT('Ctrl Pts',(-0.19068103897547,0.239358210205861,
0.0657064966754378));
#31837=CARTESIAN_POINT('Ctrl Pts',(-0.275669308368296,0.132968726389537,
0.0711207302467392));
#31838=CARTESIAN_POINT('Ctrl Pts',(-0.300900441972001,0.0222585036177047,
0.0756307716387691));
#31839=CARTESIAN_POINT('Ctrl Pts',(-0.292110160241601,-0.0551960737139081,
0.0787875627319099));
#31840=CARTESIAN_POINT('Ctrl Pts',(-0.279833018161878,-0.0977913812013095,
0.0805913361942464));
#31841=CARTESIAN_POINT('Ctrl Pts',(-0.248799516171456,-0.172907063390399,
0.0838980938896731));
#31842=CARTESIAN_POINT('Ctrl Pts',(-0.157090879780932,-0.271919338836937,
0.0891579601221785));
#31843=CARTESIAN_POINT('Ctrl Pts',(0.023450493308891,-0.312990434018135,
0.0963707260335879));
#31844=CARTESIAN_POINT('Ctrl Pts',(0.18131798103562,-0.25106041949659,0.102981727384833));
#31845=CARTESIAN_POINT('Ctrl Pts',(0.275476413276219,-0.132616711396579,
0.108991757135753));
#31846=CARTESIAN_POINT('Ctrl Pts',(0.305859403306453,1.75294825909618E-5,
0.114400912598483));
#31847=CARTESIAN_POINT('Ctrl Pts',(0.275488262452244,0.132749583053741,
0.11981042719508));
#31848=CARTESIAN_POINT('Ctrl Pts',(0.190657413586372,0.239219379063661,
0.125220540905927));
#31849=CARTESIAN_POINT('Ctrl Pts',(0.0679580198860075,0.298252809245818,
0.130631420428721));
#31850=CARTESIAN_POINT('Ctrl Pts',(-0.0682628639615764,0.298299872442762,
0.136043298037454));
#31851=CARTESIAN_POINT('Ctrl Pts',(-0.190903109853683,0.239181080607407,
0.141456373034151));
#31852=CARTESIAN_POINT('Ctrl Pts',(-0.276065680943723,0.132593720175959,
0.146870863206197));
#31853=CARTESIAN_POINT('Ctrl Pts',(-0.306004572638831,-7.02355279394243E-5,
0.15228698901937));
#31854=CARTESIAN_POINT('Ctrl Pts',(-0.266572495720376,-0.177966792725148,
0.159510876102804));
#31855=CARTESIAN_POINT('Ctrl Pts',(-0.0755420141437979,-0.330844040968773,
0.168545866717772));
#31856=CARTESIAN_POINT('Ctrl Pts',(0.212146858309987,-0.265560948222135,
0.179397548526666));
#31857=CARTESIAN_POINT('Ctrl Pts',(0.340075411028669,0.000609232641378717,
0.19026070926692));
#31858=CARTESIAN_POINT('Ctrl Pts',(0.233301287065815,0.221612007646323,
0.199324114439432));
#31859=CARTESIAN_POINT('Ctrl Pts',(0.0678658260526744,0.300036005250322,
0.206582184805351));
#31860=CARTESIAN_POINT('Ctrl Pts',(-0.0689173179449983,0.300383347622569,
0.212029566572711));
#31861=CARTESIAN_POINT('Ctrl Pts',(-0.1926289646447,0.240684814109104,0.217480994418533));
#31862=CARTESIAN_POINT('Ctrl Pts',(-0.278235295212214,0.133447490935984,
0.222936674155516));
#31863=CARTESIAN_POINT('Ctrl Pts',(-0.30878671001653,-0.000548565157992426,
0.228396798149705));
#31864=CARTESIAN_POINT('Ctrl Pts',(-0.278253232166184,-0.13463029520536,
0.233861524378761));
#31865=CARTESIAN_POINT('Ctrl Pts',(-0.192405461785685,-0.242206618549997,
0.239331056898387));
#31866=CARTESIAN_POINT('Ctrl Pts',(-0.0683064866778343,-0.302069560502724,
0.244805628557127));
#31867=CARTESIAN_POINT('Ctrl Pts',(0.0695574987923262,-0.301984756295867,
0.250285393496364));
#31868=CARTESIAN_POINT('Ctrl Pts',(0.207841992242269,-0.235606303949781,
0.25637992006153));
#31869=CARTESIAN_POINT('Ctrl Pts',(0.304940375421062,-0.0934010154145467,
0.26309199604083));
#31870=CARTESIAN_POINT('Ctrl Pts',(0.305076348451544,0.0948036199515923,
0.270424418777817));
#31871=CARTESIAN_POINT('Ctrl Pts',(0.198835199181958,0.25050195808659,0.277767683891008));
#31872=CARTESIAN_POINT('Ctrl Pts',(0.0232685326754069,0.319598579521238,
0.285122049639541));
#31873=CARTESIAN_POINT('Ctrl Pts',(-0.161163670412757,0.277517849683546,
0.292488048692369));
#31874=CARTESIAN_POINT('Ctrl Pts',(-0.279108455532343,0.150266199480721,
0.299251126448657));
#31875=CARTESIAN_POINT('Ctrl Pts',(-0.313444344793882,-0.00084859398882846,
0.305408493993884));
#31876=CARTESIAN_POINT('Ctrl Pts',(-0.282505268282257,-0.137014310816318,
0.310956928179577));
#31877=CARTESIAN_POINT('Ctrl Pts',(-0.195261921712917,-0.246230960103103,
0.316513236752478));
#31878=CARTESIAN_POINT('Ctrl Pts',(-0.0692111802430976,-0.307213573846843,
0.322075524046817));
#31879=CARTESIAN_POINT('Ctrl Pts',(0.0710557555603892,-0.306861663537198,
0.327648701198013));
#31880=CARTESIAN_POINT('Ctrl Pts',(0.197474063293807,-0.246618398330353,
0.333224270871386));
#31881=CARTESIAN_POINT('Ctrl Pts',(0.285319369726677,-0.135402277387047,
0.338817890656192));
#31882=CARTESIAN_POINT('Ctrl Pts',(0.305907629221196,-0.0462097653749184,
0.342535764331766));
#31883=CARTESIAN_POINT('Ctrl Pts',(0.306078438298251,0.00106222211004659,
0.344411755539274));
#31884=CARTESIAN_POINT('Ctrl Pts',(0.315101647298455,-0.00128170895505734,
0.0619405265894516));
#31885=CARTESIAN_POINT('Ctrl Pts',(0.31492625461718,0.0472588065417078,
0.0638668593942953));
#31886=CARTESIAN_POINT('Ctrl Pts',(0.293727533658683,0.139191100388604,
0.0676985669032832));
#31887=CARTESIAN_POINT('Ctrl Pts',(0.203343654855236,0.253543873366989,
0.073451247670091));
#31888=CARTESIAN_POINT('Ctrl Pts',(0.0733096721848766,0.315539064523512,
0.0791872665185006));
#31889=CARTESIAN_POINT('Ctrl Pts',(-0.0708947358221901,0.315877322819963,
0.0849167160876448));
#31890=CARTESIAN_POINT('Ctrl Pts',(-0.200459890912327,0.253197165795973,
0.0906340723155647));
#31891=CARTESIAN_POINT('Ctrl Pts',(-0.290049959442992,0.140992188597427,
0.0963425721181722));
#31892=CARTESIAN_POINT('Ctrl Pts',(-0.316598605249467,0.0244332032193379,
0.101091233310832));
#31893=CARTESIAN_POINT('Ctrl Pts',(-0.307350474919786,-0.0570254397486972,
0.104411192517556));
#31894=CARTESIAN_POINT('Ctrl Pts',(-0.294446049587025,-0.101795700206291,
0.10630710240828));
#31895=CARTESIAN_POINT('Ctrl Pts',(-0.261838458042338,-0.180719311846423,
0.109781473180646));
#31896=CARTESIAN_POINT('Ctrl Pts',(-0.165560810784372,-0.284601056523487,
0.115301664113939));
#31897=CARTESIAN_POINT('Ctrl Pts',(0.0235312279036465,-0.327555783312208,
0.122855538346143));
#31898=CARTESIAN_POINT('Ctrl Pts',(0.188503486018219,-0.262779385929021,
0.129764974303623));
#31899=CARTESIAN_POINT('Ctrl Pts',(0.286705132748725,-0.139203688799005,
0.136034616453424));
#31900=CARTESIAN_POINT('Ctrl Pts',(0.318325171185559,-0.00105509771065233,
0.141668412008706));
#31901=CARTESIAN_POINT('Ctrl Pts',(0.286719151798664,0.136958826184427,
0.14729347124296));
#31902=CARTESIAN_POINT('Ctrl Pts',(0.198632022686421,0.247473183495014,
0.152909932970554));
#31903=CARTESIAN_POINT('Ctrl Pts',(0.0714522871931054,0.308633723483916,
0.158517935270725));
#31904=CARTESIAN_POINT('Ctrl Pts',(-0.0694953492578695,0.308655272195571,
0.164117604325348));
#31905=CARTESIAN_POINT('Ctrl Pts',(-0.196166722112865,0.247565229485892,
0.169709114510168));
#31906=CARTESIAN_POINT('Ctrl Pts',(-0.283964270870719,0.137632576727079,
0.175292584482011));
#31907=CARTESIAN_POINT('Ctrl Pts',(-0.31476265528893,0.00106015217748537,
0.180868211582949));
#31908=CARTESIAN_POINT('Ctrl Pts',(-0.274193925446901,-0.181763087900732,
0.188292028653664));
#31909=CARTESIAN_POINT('Ctrl Pts',(-0.0782674021616253,-0.338319258809273,
0.197552960595143));
#31910=CARTESIAN_POINT('Ctrl Pts',(0.21553531409664,-0.271395910669738,
0.208637010915907));
#31911=CARTESIAN_POINT('Ctrl Pts',(0.345513151112905,-0.00038789181246443,
0.219693495439871));
#31912=CARTESIAN_POINT('Ctrl Pts',(0.237056710850022,0.223658672152894,
0.228885208413172));
#31913=CARTESIAN_POINT('Ctrl Pts',(0.0697234149934862,0.302932208439939,
0.236226210010088));
#31914=CARTESIAN_POINT('Ctrl Pts',(-0.0683760040706116,0.303260211496953,
0.241725864636005));
#31915=CARTESIAN_POINT('Ctrl Pts',(-0.19303555845014,0.243069649037974,
0.247219669375935));
#31916=CARTESIAN_POINT('Ctrl Pts',(-0.27913043167095,0.135177892286265,
0.252707771531946));
#31917=CARTESIAN_POINT('Ctrl Pts',(-0.309779544180159,0.000622981248504958,
0.258190394873152));
#31918=CARTESIAN_POINT('Ctrl Pts',(-0.279149094048921,-0.133761341722244,
0.263667655624343));
#31919=CARTESIAN_POINT('Ctrl Pts',(-0.193238240682731,-0.241370806381079,
0.269139780151241));
#31920=CARTESIAN_POINT('Ctrl Pts',(-0.0692929091135377,-0.301128915488362,
0.274606991419976));
#31921=CARTESIAN_POINT('Ctrl Pts',(0.0681349598665013,-0.301016236101523,
0.2800694292738));
#31922=CARTESIAN_POINT('Ctrl Pts',(0.205722480619705,-0.234937901808181,
0.286133732978082));
#31923=CARTESIAN_POINT('Ctrl Pts',(0.302082544121992,-0.093704256729346,
0.292798181344527));
#31924=CARTESIAN_POINT('Ctrl Pts',(0.302150472949551,0.0927223497626265,
0.300061261848913));
#31925=CARTESIAN_POINT('Ctrl Pts',(0.19711290358951,0.246534520123679,0.307317361175983));
#31926=CARTESIAN_POINT('Ctrl Pts',(0.024014651371324,0.314590469125311,
0.314567245913451));
#31927=CARTESIAN_POINT('Ctrl Pts',(-0.157345516009493,0.273139119421548,
0.321811112240196));
#31928=CARTESIAN_POINT('Ctrl Pts',(-0.273017499230799,0.148255125916073,
0.328446171918567));
#31929=CARTESIAN_POINT('Ctrl Pts',(-0.306603925817584,0.000295637397937573,
0.334474828088449));
#31930=CARTESIAN_POINT('Ctrl Pts',(-0.276342099141224,-0.132785077310565,
0.339897459977899));
#31931=CARTESIAN_POINT('Ctrl Pts',(-0.191200427627164,-0.239318641719874,
0.345318556602232));
#31932=CARTESIAN_POINT('Ctrl Pts',(-0.0684258001418649,-0.298703158508728,
0.350735481649343));
#31933=CARTESIAN_POINT('Ctrl Pts',(0.0679566655576182,-0.298312240153081,
0.356154839923386));
#31934=CARTESIAN_POINT('Ctrl Pts',(0.190650317768282,-0.239856073740776,
0.361565262555767));
#31935=CARTESIAN_POINT('Ctrl Pts',(0.275745802382817,-0.131995078166987,
0.366987994062727));
#31936=CARTESIAN_POINT('Ctrl Pts',(0.295638197983241,-0.045872517774112,
0.370578103976212));
#31937=CARTESIAN_POINT('Ctrl Pts',(0.295803909517168,-1.12925223861182E-5,
0.372398109013342));
#31938=CARTESIAN_POINT('Ctrl Pts',(0.344894607025859,-0.00117220091143172,
0.0618937486917298));
#31939=CARTESIAN_POINT('Ctrl Pts',(0.344703966040985,0.051588333982661,
0.0639875531791247));
#31940=CARTESIAN_POINT('Ctrl Pts',(0.321489911562902,0.152620094193498,
0.0681973923342701));
#31941=CARTESIAN_POINT('Ctrl Pts',(0.22256664720873,0.277542883006417,0.0744854517154489));
#31942=CARTESIAN_POINT('Ctrl Pts',(0.0802116976126469,0.345540567216692,
0.0807688522723124));
#31943=CARTESIAN_POINT('Ctrl Pts',(-0.0776391716305396,0.345840974720998,
0.087038807205936));
#31944=CARTESIAN_POINT('Ctrl Pts',(-0.219508915025033,0.277260432316066,
0.0932998185216175));
#31945=CARTESIAN_POINT('Ctrl Pts',(-0.317591755286808,0.154390861205383,
0.0995493368234934));
#31946=CARTESIAN_POINT('Ctrl Pts',(-0.346661039759245,0.0267922753448241,
0.104748509576963));
#31947=CARTESIAN_POINT('Ctrl Pts',(-0.336535485770271,-0.0623898119372897,
0.108383100293887));
#31948=CARTESIAN_POINT('Ctrl Pts',(-0.322408424731889,-0.111401720018576,
0.110458667643685));
#31949=CARTESIAN_POINT('Ctrl Pts',(-0.286711444159767,-0.197802933078996,
0.114262205448296));
#31950=CARTESIAN_POINT('Ctrl Pts',(-0.181320545975211,-0.311512954024223,
0.120304748022494));
#31951=CARTESIAN_POINT('Ctrl Pts',(0.0256366134017508,-0.358518960303294,
0.128572221561375));
#31952=CARTESIAN_POINT('Ctrl Pts',(0.206149878169194,-0.287632860671769,
0.136132629991281));
#31953=CARTESIAN_POINT('Ctrl Pts',(0.313573318790257,-0.152444007237616,
0.142991291085792));
#31954=CARTESIAN_POINT('Ctrl Pts',(0.348151986684333,-0.00135155530985844,
0.149152888630487));
#31955=CARTESIAN_POINT('Ctrl Pts',(0.313588656288107,0.14954981179416,0.155303241992947));
#31956=CARTESIAN_POINT('Ctrl Pts',(0.217300641502055,0.270344572766772,
0.161442322103795));
#31957=CARTESIAN_POINT('Ctrl Pts',(0.0783302437237461,0.33716785546378,
0.167570083359719));
#31958=CARTESIAN_POINT('Ctrl Pts',(-0.0756245191684134,0.337184670947358,
0.173686512217792));
#31959=CARTESIAN_POINT('Ctrl Pts',(-0.213926786047297,0.270477291973825,
0.179791561237685));
#31960=CARTESIAN_POINT('Ctrl Pts',(-0.309740427769701,0.150493872976662,
0.185885228264861));
#31961=CARTESIAN_POINT('Ctrl Pts',(-0.3433301135152,0.00151097286038558,
0.191967471988919));
#31962=CARTESIAN_POINT('Ctrl Pts',(-0.299082473709324,-0.197828041114981,
0.200061909718623));
#31963=CARTESIAN_POINT('Ctrl Pts',(-0.0855849665151933,-0.368340181506443,
0.210151340739428));
#31964=CARTESIAN_POINT('Ctrl Pts',(0.234108819111557,-0.295422317233866,
0.222212862825778));
#31965=CARTESIAN_POINT('Ctrl Pts',(0.375268601750312,-0.000857533008588078,
0.234228580964883));
#31966=CARTESIAN_POINT('Ctrl Pts',(0.25749264156393,0.242240410083148,0.24420359765261));
#31967=CARTESIAN_POINT('Ctrl Pts',(0.076109197473031,0.328146093635365,
0.252160795683558));
#31968=CARTESIAN_POINT('Ctrl Pts',(-0.0734630576993165,0.328488983850561,
0.258117334003062));
#31969=CARTESIAN_POINT('Ctrl Pts',(-0.208357730141545,0.263339735952782,
0.264062515706671));
#31970=CARTESIAN_POINT('Ctrl Pts',(-0.301433211455292,0.146675275774542,
0.269996393190013));
#31971=CARTESIAN_POINT('Ctrl Pts',(-0.334527391943304,0.00131958428967035,
0.275918982746397));
#31972=CARTESIAN_POINT('Ctrl Pts',(-0.30145311065115,-0.143710382389741,
0.281830329757323));
#31973=CARTESIAN_POINT('Ctrl Pts',(-0.208811314453104,-0.25972617686706,
0.287730466702406));
#31974=CARTESIAN_POINT('Ctrl Pts',(-0.0752963160901684,-0.324078250133092,
0.293619451824586));
#31975=CARTESIAN_POINT('Ctrl Pts',(0.0725822231329485,-0.323940922408941,
0.299497337556348));
#31976=CARTESIAN_POINT('Ctrl Pts',(0.220469193575753,-0.252893157585676,
0.306015977608672));
#31977=CARTESIAN_POINT('Ctrl Pts',(0.323888963496138,-0.101243997194457,
0.313170937392681));
#31978=CARTESIAN_POINT('Ctrl Pts',(0.323914718356231,0.0986015513486016,
0.320956782079779));
#31979=CARTESIAN_POINT('Ctrl Pts',(0.211450301619867,0.263207970933167,
0.328723492520748));
#31980=CARTESIAN_POINT('Ctrl Pts',(0.0264517346568824,0.335890378755159,
0.336471005872168));
#31981=CARTESIAN_POINT('Ctrl Pts',(-0.167033447139801,0.291616636207715,
0.344199700797049));
#31982=CARTESIAN_POINT('Ctrl Pts',(-0.290203018169231,0.158568415055973,
0.35126714050295));
#31983=CARTESIAN_POINT('Ctrl Pts',(-0.325900520055194,0.00120617226061592,
0.35767858494089));
#31984=CARTESIAN_POINT('Ctrl Pts',(-0.29373299888089,-0.140130990161181,
0.363438374653413));
#31985=CARTESIAN_POINT('Ctrl Pts',(-0.203410557114407,-0.253129387443769,
0.369188308457246));
#31986=CARTESIAN_POINT('Ctrl Pts',(-0.0733398244589557,-0.315984228529682,
0.374927114369164));
#31987=CARTESIAN_POINT('Ctrl Pts',(0.070907119541957,-0.315592776376067,
0.380658098012618));
#31988=CARTESIAN_POINT('Ctrl Pts',(0.200499120082281,-0.253747220752294,
0.386375419790931));
#31989=CARTESIAN_POINT('Ctrl Pts',(0.290231966152725,-0.14011003674842,
0.392090289367516));
#31990=CARTESIAN_POINT('Ctrl Pts',(0.311180051930582,-0.0491735403917148,
0.395880310107509));
#31991=CARTESIAN_POINT('Ctrl Pts',(0.311353847170781,-0.00107512219721069,
0.397789098259406));
#31992=CARTESIAN_POINT('Ctrl Pts',(0.36349947386268,-0.000182513280454622,
0.0386491721592961));
#31993=CARTESIAN_POINT('Ctrl Pts',(0.363299197931637,0.0552445254292098,
0.0408487969850539));
#31994=CARTESIAN_POINT('Ctrl Pts',(0.338822849801048,0.162017987113332,
0.0452971626933041));
#31995=CARTESIAN_POINT('Ctrl Pts',(0.234401841864732,0.293778560944321,
0.0519311472688644));
#31996=CARTESIAN_POINT('Ctrl Pts',(0.0839251224276196,0.365759381145584,
0.0585757604749919));
#31997=CARTESIAN_POINT('Ctrl Pts',(-0.0831258602463933,0.366054544758465,
0.0652102611487041));
#31998=CARTESIAN_POINT('Ctrl Pts',(-0.233480113083901,0.293431779736776,
0.0718457140698859));
#31999=CARTESIAN_POINT('Ctrl Pts',(-0.337548697207091,0.163079909212871,
0.0784755564546323));
#32000=CARTESIAN_POINT('Ctrl Pts',(-0.368445531345481,0.0275650217023474,
0.0839980235483959));
#32001=CARTESIAN_POINT('Ctrl Pts',(-0.357684839286351,-0.0672426651280164,
0.0878617768994511));
#32002=CARTESIAN_POINT('Ctrl Pts',(-0.342661576869175,-0.119365372087535,
0.0900691038896605));
#32003=CARTESIAN_POINT('Ctrl Pts',(-0.304688860407797,-0.211277600934222,
0.0941152586155943));
#32004=CARTESIAN_POINT('Ctrl Pts',(-0.192498270408811,-0.332377332372952,
0.100549392864518));
#32005=CARTESIAN_POINT('Ctrl Pts',(0.0281733882059037,-0.382550621286202,
0.109365111791553));
#32006=CARTESIAN_POINT('Ctrl Pts',(0.220954062612933,-0.306893333992967,
0.11743876178892));
#32007=CARTESIAN_POINT('Ctrl Pts',(0.335829202294293,-0.162364653417003,
0.12477195777997));
#32008=CARTESIAN_POINT('Ctrl Pts',(0.372856255837749,-0.000655007332560676,
0.131366750230641));
#32009=CARTESIAN_POINT('Ctrl Pts',(0.335844870938437,0.161025293563643,
0.137956255408633));
#32010=CARTESIAN_POINT('Ctrl Pts',(0.232592962625393,0.290584863175236,
0.144540250872817));
#32011=CARTESIAN_POINT('Ctrl Pts',(0.0834124279892051,0.362339037782258,
0.151118603972318));
#32012=CARTESIAN_POINT('Ctrl Pts',(-0.0820214421351618,0.362374494803792,
0.157691097018862));
#32013=CARTESIAN_POINT('Ctrl Pts',(-0.230783736935749,0.290641660029172,
0.164257575225425));
#32014=CARTESIAN_POINT('Ctrl Pts',(-0.333948068275454,0.161482550546205,
0.170817836066568));
#32015=CARTESIAN_POINT('Ctrl Pts',(-0.370156587532269,0.00094904835990728,
0.17737170980749));
#32016=CARTESIAN_POINT('Ctrl Pts',(-0.322463302031498,-0.214034687891742,
0.186101501609228));
#32017=CARTESIAN_POINT('Ctrl Pts',(-0.0919790405353035,-0.398250109605909,
0.196996893196212));
#32018=CARTESIAN_POINT('Ctrl Pts',(0.253842468120618,-0.31950787991112,
0.210043175686943));
#32019=CARTESIAN_POINT('Ctrl Pts',(0.406874486079669,-0.000451865866853843,
0.223059865384761));
#32020=CARTESIAN_POINT('Ctrl Pts',(0.27918181167757,0.263318543608872,0.233881466919701));
#32021=CARTESIAN_POINT('Ctrl Pts',(0.0822068433707472,0.356629457468139,
0.242522733897225));
#32022=CARTESIAN_POINT('Ctrl Pts',(-0.0803281279023186,0.357012622815529,
0.248995529534002));
#32023=CARTESIAN_POINT('Ctrl Pts',(-0.227011595006363,0.286182978182527,
0.255460035897147));
#32024=CARTESIAN_POINT('Ctrl Pts',(-0.3282873008575,0.159258591210816,0.261916079613041));
#32025=CARTESIAN_POINT('Ctrl Pts',(-0.364323816221617,0.00102235932660949,
0.268363542385575));
#32026=CARTESIAN_POINT('Ctrl Pts',(-0.3283094791852,-0.156949994186001,
0.274802294072678));
#32027=CARTESIAN_POINT('Ctrl Pts',(-0.227355336560919,-0.283388629159677,
0.281232202828533));
#32028=CARTESIAN_POINT('Ctrl Pts',(-0.081784357592912,-0.353562500688594,
0.287653104245323));
#32029=CARTESIAN_POINT('Ctrl Pts',(0.0795279050014283,-0.353420115671001,
0.294064881104805));
#32030=CARTESIAN_POINT('Ctrl Pts',(0.24092584464248,-0.275891982678635,
0.301178909350928));
#32031=CARTESIAN_POINT('Ctrl Pts',(0.353854516025502,-0.110325647039583,
0.30899075718887));
#32032=CARTESIAN_POINT('Ctrl Pts',(0.353900252047577,0.107988317536177,
0.317496095092339));
#32033=CARTESIAN_POINT('Ctrl Pts',(0.231000709833199,0.287889843051827,
0.325984040679209));
#32034=CARTESIAN_POINT('Ctrl Pts',(0.028738633598124,0.367371051552907,
0.334454691554125));
#32035=CARTESIAN_POINT('Ctrl Pts',(-0.182879793494325,0.318956105318771,
0.342907496943029));
#32036=CARTESIAN_POINT('Ctrl Pts',(-0.317637558246171,0.173408698249264,
0.35063943767884));
#32037=CARTESIAN_POINT('Ctrl Pts',(-0.356704898032242,0.00120299507430483,
0.357655313472524));
#32038=CARTESIAN_POINT('Ctrl Pts',(-0.321499156165066,-0.153473689430544,
0.36395936824658));
#32039=CARTESIAN_POINT('Ctrl Pts',(-0.222637917146764,-0.277180768652223,
0.370252746171281));
#32040=CARTESIAN_POINT('Ctrl Pts',(-0.0802353799449259,-0.34594748560465,
0.376536355268848));
#32041=CARTESIAN_POINT('Ctrl Pts',(0.0776573488015606,-0.345588985512381,
0.382807725745614));
#32042=CARTESIAN_POINT('Ctrl Pts',(0.219540463198455,-0.277752573568418,
0.389071158618383));
#32043=CARTESIAN_POINT('Ctrl Pts',(0.31776826189951,-0.153592430403837,
0.395318895203019));
#32044=CARTESIAN_POINT('Ctrl Pts',(0.340714022294167,-0.0536225369660789,
0.399484162887714));
#32045=CARTESIAN_POINT('Ctrl Pts',(0.340902966777108,-0.00133151480896985,
0.401559334739322));
#32046=CARTESIAN_POINT('Ctrl Pts',(0.356819906199823,0.000946415613638381,
0.00959378898777047));
#32047=CARTESIAN_POINT('Ctrl Pts',(0.356622877445812,0.0554747871389154,
0.0117577501610062));
#32048=CARTESIAN_POINT('Ctrl Pts',(0.332600183621965,0.16027838517997,0.0161240058481628));
#32049=CARTESIAN_POINT('Ctrl Pts',(0.229891504241292,0.289970795598527,
0.0226522300475058));
#32050=CARTESIAN_POINT('Ctrl Pts',(0.0816316084877276,0.360899492525754,
0.0291986752852052));
#32051=CARTESIAN_POINT('Ctrl Pts',(-0.0832135069240492,0.361230328558343,
0.0357458212344272));
#32052=CARTESIAN_POINT('Ctrl Pts',(-0.231812809233063,0.289476825331103,
0.0423030597446485));
#32053=CARTESIAN_POINT('Ctrl Pts',(-0.334837144696434,0.160482303310326,
0.0488649839626194));
#32054=CARTESIAN_POINT('Ctrl Pts',(-0.365483778755952,0.0261595762945765,
0.0543388585149657));
#32055=CARTESIAN_POINT('Ctrl Pts',(-0.354809005945464,-0.0679232502424184,
0.0581730130440929));
#32056=CARTESIAN_POINT('Ctrl Pts',(-0.33989224429653,-0.119677976039048,
0.060364734388816));
#32057=CARTESIAN_POINT('Ctrl Pts',(-0.302175059373086,-0.210974138360163,
0.0643837854119232));
#32058=CARTESIAN_POINT('Ctrl Pts',(-0.190646477540233,-0.331431753764648,
0.0707818924680168));
#32059=CARTESIAN_POINT('Ctrl Pts',(0.0292333963704387,-0.381494309464949,
0.079566523525864));
#32060=CARTESIAN_POINT('Ctrl Pts',(0.221739847035907,-0.306010819130579,
0.0876276515973482));
#32061=CARTESIAN_POINT('Ctrl Pts',(0.336666969672357,-0.161466621254631,
0.0949624750012229));
#32062=CARTESIAN_POINT('Ctrl Pts',(0.373785362338973,0.00051619079835515,
0.101568677763791));
#32063=CARTESIAN_POINT('Ctrl Pts',(0.336680450911145,0.162727630812525,
0.108179512361388));
#32064=CARTESIAN_POINT('Ctrl Pts',(0.232959901261762,0.292920760014865,
0.114794818884824));
#32065=CARTESIAN_POINT('Ctrl Pts',(0.0828555793888438,0.365149362703125,
0.121414368594224));
#32066=CARTESIAN_POINT('Ctrl Pts',(-0.083865947059046,0.365213561638823,
0.12803802907686));
#32067=CARTESIAN_POINT('Ctrl Pts',(-0.234022832658805,0.292837641030661,
0.134665525254689));
#32068=CARTESIAN_POINT('Ctrl Pts',(-0.33832626279477,0.162301257816034,
0.141296736338365));
#32069=CARTESIAN_POINT('Ctrl Pts',(-0.375003870302502,-0.000208826488397771,
0.147931370051417));
#32070=CARTESIAN_POINT('Ctrl Pts',(-0.326697030597439,-0.218164466286065,
0.156781999918125));
#32071=CARTESIAN_POINT('Ctrl Pts',(-0.0926206709582978,-0.405493959958885,
0.16785291225016));
#32072=CARTESIAN_POINT('Ctrl Pts',(0.25986200463863,-0.325488471750001,
0.181148799941241));
#32073=CARTESIAN_POINT('Ctrl Pts',(0.416506452243591,0.000529987086060091,
0.194453598323448));
#32074=CARTESIAN_POINT('Ctrl Pts',(0.285769963163853,0.271011892920662,
0.205547313860392));
#32075=CARTESIAN_POINT('Ctrl Pts',(0.0834145480806414,0.36692060144113,
0.214424950674681));
#32076=CARTESIAN_POINT('Ctrl Pts',(-0.0838047257248785,0.367335044836678,
0.221084512436662));
#32077=CARTESIAN_POINT('Ctrl Pts',(-0.23494910883256,0.294385829432161,
0.227745038970719));
#32078=CARTESIAN_POINT('Ctrl Pts',(-0.339462559196761,0.163440857085512,
0.234406421306329));
#32079=CARTESIAN_POINT('Ctrl Pts',(-0.376725781361808,-5.13357953542337E-5,
0.241068351157357));
#32080=CARTESIAN_POINT('Ctrl Pts',(-0.33948423973855,-0.163512941907327,
0.247730736309198));
#32081=CARTESIAN_POINT('Ctrl Pts',(-0.234900593046164,-0.29454293296101,
0.254393296337443));
#32082=CARTESIAN_POINT('Ctrl Pts',(-0.0838651541636832,-0.367377563231161,
0.261055777814004));
#32083=CARTESIAN_POINT('Ctrl Pts',(0.0837481144633832,-0.367257140719985,
0.26771807786542));
#32084=CARTESIAN_POINT('Ctrl Pts',(0.251686188309771,-0.286617551856353,
0.275119988445193));
#32085=CARTESIAN_POINT('Ctrl Pts',(0.369425843626467,-0.114101792621121,
0.283261579477833));
#32086=CARTESIAN_POINT('Ctrl Pts',(0.369531467939292,0.113815416132859,
0.292141139676902));
#32087=CARTESIAN_POINT('Ctrl Pts',(0.241042524053221,0.302013576838691,
0.30101906641207));
#32088=CARTESIAN_POINT('Ctrl Pts',(0.0291543790867535,0.385335872444532,
0.309893811897827));
#32089=CARTESIAN_POINT('Ctrl Pts',(-0.192967827991779,0.334584308776725,
0.31876582586576));
#32090=CARTESIAN_POINT('Ctrl Pts',(-0.334683709406543,0.181589938324689,
0.326895446945865));
#32091=CARTESIAN_POINT('Ctrl Pts',(-0.375847011475061,0.000280941035022615,
0.334282274883861));
#32092=CARTESIAN_POINT('Ctrl Pts',(-0.338747168017924,-0.162782317242193,
0.340928662116343));
#32093=CARTESIAN_POINT('Ctrl Pts',(-0.234418175086977,-0.293389546598337,
0.347571447558357));
#32094=CARTESIAN_POINT('Ctrl Pts',(-0.0839196627329805,-0.36605477155107,
0.354213275470552));
#32095=CARTESIAN_POINT('Ctrl Pts',(0.0831384568783626,-0.365745988360452,
0.360847755809616));
#32096=CARTESIAN_POINT('Ctrl Pts',(0.23345413252389,-0.293818325122263,
0.367485688540575));
#32097=CARTESIAN_POINT('Ctrl Pts',(0.337659987033965,-0.162302327276991,
0.374107097871543));
#32098=CARTESIAN_POINT('Ctrl Pts',(0.362055097124151,-0.0558590500639481,
0.378541577281661));
#32099=CARTESIAN_POINT('Ctrl Pts',(0.362254830155579,-0.000582260769330227,
0.380735239452708));
#32100=CARTESIAN_POINT('Ctrl Pts',(0.338971622004564,0.00122203251932272,
0.00102359537366932));
#32101=CARTESIAN_POINT('Ctrl Pts',(0.338783697626477,0.0532307373322113,
0.00308756344638532));
#32102=CARTESIAN_POINT('Ctrl Pts',(0.315964718113649,0.152606406913278,
0.00722828744846333));
#32103=CARTESIAN_POINT('Ctrl Pts',(0.218309382196408,0.276052874201225,
0.0134401453573786));
#32104=CARTESIAN_POINT('Ctrl Pts',(0.0772757052457959,0.343472830879594,
0.0196657590309892));
#32105=CARTESIAN_POINT('Ctrl Pts',(-0.0796437906546839,0.343832157897091,
0.0258990935001355));
#32106=CARTESIAN_POINT('Ctrl Pts',(-0.221168105741207,0.275483129904846,
0.0321436146842611));
#32107=CARTESIAN_POINT('Ctrl Pts',(-0.319355815536309,0.1525741006545,0.0383970939432339));
#32108=CARTESIAN_POINT('Ctrl Pts',(-0.348587348280596,0.024487125389868,
0.0436166583023114));
#32109=CARTESIAN_POINT('Ctrl Pts',(-0.338406476397144,-0.0652656093556688,
0.0472744271625356));
#32110=CARTESIAN_POINT('Ctrl Pts',(-0.324173395788412,-0.114649375725035,
0.0493657286531609));
#32111=CARTESIAN_POINT('Ctrl Pts',(-0.28817943011689,-0.201776041439395,
0.0532012486093371));
#32112=CARTESIAN_POINT('Ctrl Pts',(-0.181699334707641,-0.31681173755523,
0.0593107734350504));
#32113=CARTESIAN_POINT('Ctrl Pts',(0.0284239805984007,-0.364683407763082,
0.067705875653049));
#32114=CARTESIAN_POINT('Ctrl Pts',(0.212569436660183,-0.292507310629878,
0.0754165362004278));
#32115=CARTESIAN_POINT('Ctrl Pts',(0.322599477836521,-0.15414718734826,
0.0824380381498116));
#32116=CARTESIAN_POINT('Ctrl Pts',(0.358168918258642,0.00101965913172981,
0.0887663839950056));
#32117=CARTESIAN_POINT('Ctrl Pts',(0.322612964209937,0.156522586796577,
0.0951037160190564));
#32118=CARTESIAN_POINT('Ctrl Pts',(0.223123755288736,0.281426747319146,
0.10144980766624));
#32119=CARTESIAN_POINT('Ctrl Pts',(0.0790274718456132,0.350779549406656,
0.107804689616852));
#32120=CARTESIAN_POINT('Ctrl Pts',(-0.0811457239354608,0.350856478590949,
0.114168132635694));
#32121=CARTESIAN_POINT('Ctrl Pts',(-0.225519703943384,0.281282412546895,
0.120540137083061));
#32122=CARTESIAN_POINT('Ctrl Pts',(-0.325891610114915,0.155693758731515,
0.126920496791768));
#32123=CARTESIAN_POINT('Ctrl Pts',(-0.36122095909014,-0.000791144434539592,
0.13330915705397));
#32124=CARTESIAN_POINT('Ctrl Pts',(-0.314693637784338,-0.210830847787741,
0.141838312536158));
#32125=CARTESIAN_POINT('Ctrl Pts',(-0.0889149329510122,-0.391648089547769,
0.15251966736754));
#32126=CARTESIAN_POINT('Ctrl Pts',(0.251752009513806,-0.314464296529647,
0.165368610987597));
#32127=CARTESIAN_POINT('Ctrl Pts',(0.403510758968937,0.00106941916421913,
0.178247703836957));
#32128=CARTESIAN_POINT('Ctrl Pts',(0.276843416708589,0.263393027280319,
0.189004268698655));
#32129=CARTESIAN_POINT('Ctrl Pts',(0.0803728550066286,0.356538695494576,
0.197623801156164));
#32130=CARTESIAN_POINT('Ctrl Pts',(-0.082124722949435,0.356960248773731,
0.20409515149567));
#32131=CARTESIAN_POINT('Ctrl Pts',(-0.229138298513218,0.286019839365132,
0.210573278023524));
#32132=CARTESIAN_POINT('Ctrl Pts',(-0.330899321428319,0.158559897907127,
0.217057866538153));
#32133=CARTESIAN_POINT('Ctrl Pts',(-0.367218419527253,-0.00073938524378964,
0.223548897362093));
#32134=CARTESIAN_POINT('Ctrl Pts',(-0.330922063223575,-0.160159900840358,
0.230046159510642));
#32135=CARTESIAN_POINT('Ctrl Pts',(-0.228842222130787,-0.288070568178848,
0.236549534276728));
#32136=CARTESIAN_POINT('Ctrl Pts',(-0.081285433209043,-0.359253201003627,
0.243058873820311));
#32137=CARTESIAN_POINT('Ctrl Pts',(0.0826297065064189,-0.359147357935786,
0.249573876443222));
#32138=CARTESIAN_POINT('Ctrl Pts',(0.247033301398344,-0.280231436867822,
0.256819508059951));
#32139=CARTESIAN_POINT('Ctrl Pts',(0.362424113255112,-0.111212706412119,
0.264796306809896));
#32140=CARTESIAN_POINT('Ctrl Pts',(0.362579145870285,0.112420181971907,
0.273508907247649));
#32141=CARTESIAN_POINT('Ctrl Pts',(0.236388248958002,0.297313675401446,
0.282229310951794));
#32142=CARTESIAN_POINT('Ctrl Pts',(0.0279736069790582,0.379327219628356,
0.290959274341561));
#32143=CARTESIAN_POINT('Ctrl Pts',(-0.190797195609782,0.329377211540027,
0.299696539230122));
#32144=CARTESIAN_POINT('Ctrl Pts',(-0.330585412823941,0.178542452477963,
0.307712637727993));
#32145=CARTESIAN_POINT('Ctrl Pts',(-0.371243104476414,-0.000474749941338493,
0.315006066901667));
#32146=CARTESIAN_POINT('Ctrl Pts',(-0.334606457675173,-0.161629723946379,
0.321573991917603));
#32147=CARTESIAN_POINT('Ctrl Pts',(-0.231407664655513,-0.290837615251207,
0.328145128710479));
#32148=CARTESIAN_POINT('Ctrl Pts',(-0.0823972989864712,-0.362820576105573,
0.334721509538079));
#32149=CARTESIAN_POINT('Ctrl Pts',(0.0831903606930065,-0.362517654622939,
0.341297320706161));
#32150=CARTESIAN_POINT('Ctrl Pts',(0.232343277189241,-0.291185914112765,
0.347883079367717));
#32151=CARTESIAN_POINT('Ctrl Pts',(0.335838209534233,-0.160562321531647,
0.354458910889608));
#32152=CARTESIAN_POINT('Ctrl Pts',(0.360088128449173,-0.0547760251224751,
0.358865946090263));
#32153=CARTESIAN_POINT('Ctrl Pts',(0.360286796917659,0.000206142791657797,
0.361047916196966));
#32154=CARTESIAN_POINT('Ctrl Pts',(0.329995701589468,0.00118959959741402,
0.00102359537366932));
#32155=CARTESIAN_POINT('Ctrl Pts',(0.329812358348379,0.0519304593106012,
0.00303724894968045));
#32156=CARTESIAN_POINT('Ctrl Pts',(0.307603150250096,0.14856309907024,0.007063921474547));
#32157=CARTESIAN_POINT('Ctrl Pts',(0.212522007054295,0.2688270154723,0.0131144005095069));
#32158=CARTESIAN_POINT('Ctrl Pts',(0.0751961041762406,0.33443845631537,
0.0191752186885983));
#32159=CARTESIAN_POINT('Ctrl Pts',(-0.0776142387319525,0.334810528053721,
0.025245738062024));
#32160=CARTESIAN_POINT('Ctrl Pts',(-0.215432226705683,0.268236493442132,
0.0313264548832147));
#32161=CARTESIAN_POINT('Ctrl Pts',(-0.311063582237146,0.148538498980413,
0.0374170400486292));
#32162=CARTESIAN_POINT('Ctrl Pts',(-0.339534702539374,0.0237758430999062,
0.0425008539245673));
#32163=CARTESIAN_POINT('Ctrl Pts',(-0.329617478537296,-0.0636510452603832,
0.0460638560210726));
#32164=CARTESIAN_POINT('Ctrl Pts',(-0.315752180564557,-0.111758567679568,
0.0481010960909614));
#32165=CARTESIAN_POINT('Ctrl Pts',(-0.280687728436729,-0.19663499457563,
0.0518375549362775));
#32166=CARTESIAN_POINT('Ctrl Pts',(-0.176953832876605,-0.308707864139412,
0.0577895429568186));
#32167=CARTESIAN_POINT('Ctrl Pts',(0.0277912542949835,-0.355359243876355,
0.0659698006169508));
#32168=CARTESIAN_POINT('Ctrl Pts',(0.207256209567046,-0.285022432777545,
0.073484386523706));
#32169=CARTESIAN_POINT('Ctrl Pts',(0.31450859302708,-0.150158997366471,
0.0803284879538114));
#32170=CARTESIAN_POINT('Ctrl Pts',(0.349186611535958,0.00111014849211965,
0.0864979120385476));
#32171=CARTESIAN_POINT('Ctrl Pts',(0.314520756767304,0.152731777144028,
0.0926770234710082));
#32172=CARTESIAN_POINT('Ctrl Pts',(0.217500483746742,0.274539465175591,
0.098865768103921));
#32173=CARTESIAN_POINT('Ctrl Pts',(0.0769551264679099,0.342186713109751,
0.105064101576398));
#32174=CARTESIAN_POINT('Ctrl Pts',(-0.0793009475509065,0.342263708237282,
0.111271969453101));
#32175=CARTESIAN_POINT('Ctrl Pts',(-0.220172034550062,0.274381760656883,
0.117489309777858));
#32176=CARTESIAN_POINT('Ctrl Pts',(-0.318128621603507,0.151819046241454,
0.123716067105663));
#32177=CARTESIAN_POINT('Ctrl Pts',(-0.352617648223723,-0.000927697002303161,
0.129952164368648));
#32178=CARTESIAN_POINT('Ctrl Pts',(-0.307197248189229,-0.205991895653557,
0.138279361997572));
#32179=CARTESIAN_POINT('Ctrl Pts',(-0.0867093646975666,-0.382606488631909,
0.148711360096893));
#32180=CARTESIAN_POINT('Ctrl Pts',(0.246157896760925,-0.307226237821677,
0.16126605881999));
#32181=CARTESIAN_POINT('Ctrl Pts',(0.394548713993526,0.00121213976701099,
0.173856329664019));
#32182=CARTESIAN_POINT('Ctrl Pts',(0.270683494680064,0.25779707362797,0.184377360469391));
#32183=CARTESIAN_POINT('Ctrl Pts',(0.0784480660104459,0.348945360245205,
0.192811248605432));
#32184=CARTESIAN_POINT('Ctrl Pts',(-0.0805931042682236,0.349358375490888,
0.199145126960344));
#32185=CARTESIAN_POINT('Ctrl Pts',(-0.224524686851408,0.279914574363962,
0.205487348255157));
#32186=CARTESIAN_POINT('Ctrl Pts',(-0.324178791380424,0.155094279198964,
0.211837815149481));
#32187=CARTESIAN_POINT('Ctrl Pts',(-0.359765231562575,-0.000950160030172512,
0.218196411362682));
#32188=CARTESIAN_POINT('Ctrl Pts',(-0.324199918380757,-0.157162565812712,
0.22456305908972));
#32189=CARTESIAN_POINT('Ctrl Pts',(-0.224151419632265,-0.282543079616346,
0.230937631934188));
#32190=CARTESIAN_POINT('Ctrl Pts',(-0.0794762745603369,-0.352337612459348,
0.237319995378052));
#32191=CARTESIAN_POINT('Ctrl Pts',(0.0812906306420514,-0.352242766117238,
0.243710053380832));
#32192=CARTESIAN_POINT('Ctrl Pts',(0.242583044989387,-0.274824345329341,
0.250818566710242));
#32193=CARTESIAN_POINT('Ctrl Pts',(0.355857692111688,-0.108936398125315,
0.258648506513342));
#32194=CARTESIAN_POINT('Ctrl Pts',(0.35601905515454,0.110643209305051,0.267203260973594));
#32195=CARTESIAN_POINT('Ctrl Pts',(0.232065828412221,0.292295611594562,
0.275770669585301));
#32196=CARTESIAN_POINT('Ctrl Pts',(0.0272435837717024,0.37290401539681,
0.284350408116761));
#32197=CARTESIAN_POINT('Ctrl Pts',(-0.187879927304316,0.323810447294939,
0.292942183858905));
#32198=CARTESIAN_POINT('Ctrl Pts',(-0.325407735789747,0.17542191209667,
0.300828814614272));
#32199=CARTESIAN_POINT('Ctrl Pts',(-0.365431318619722,-0.00075089577638709,
0.308006589851792));
#32200=CARTESIAN_POINT('Ctrl Pts',(-0.329362034481868,-0.159416832712907,
0.314473213303831));
#32201=CARTESIAN_POINT('Ctrl Pts',(-0.227729428899003,-0.286678573326201,
0.320945361203317));
#32202=CARTESIAN_POINT('Ctrl Pts',(-0.0809152203341978,-0.357609127112455,
0.327424927538347));
#32203=CARTESIAN_POINT('Ctrl Pts',(0.0823028008577847,-0.357312684079966,
0.333907107762849));
#32204=CARTESIAN_POINT('Ctrl Pts',(0.229369976399687,-0.286999416296364,
0.340400245782608));
#32205=CARTESIAN_POINT('Ctrl Pts',(0.331477217034357,-0.158117971828307,
0.346888605564388));
#32206=CARTESIAN_POINT('Ctrl Pts',(0.355417803964002,-0.0537733405890617,
0.351235961881927));
#32207=CARTESIAN_POINT('Ctrl Pts',(0.355614008397637,0.000526897379297947,
0.35339086956434));
#32208=CARTESIAN_POINT('',(0.329995701589468,0.00118959959741402,0.00102359537366932));
#32209=CARTESIAN_POINT('Origin',(0.33,2.0618100472869E-19,0.031));
#32210=CARTESIAN_POINT('',(0.355614008397637,0.000526897379297947,0.35339086956434));
#32211=CARTESIAN_POINT('Ctrl Pts',(0.329995701589468,0.00118959959741402,
0.00102359537366932));
#32212=CARTESIAN_POINT('Ctrl Pts',(0.329812358348379,0.0519304593106012,
0.00303724894968045));
#32213=CARTESIAN_POINT('Ctrl Pts',(0.307603150250096,0.14856309907024,0.007063921474547));
#32214=CARTESIAN_POINT('Ctrl Pts',(0.212522007054295,0.2688270154723,0.0131144005095069));
#32215=CARTESIAN_POINT('Ctrl Pts',(0.0751961041762406,0.33443845631537,
0.0191752186885983));
#32216=CARTESIAN_POINT('Ctrl Pts',(-0.0776142387319525,0.334810528053721,
0.025245738062024));
#32217=CARTESIAN_POINT('Ctrl Pts',(-0.215432226705683,0.268236493442132,
0.0313264548832147));
#32218=CARTESIAN_POINT('Ctrl Pts',(-0.311063582237146,0.148538498980413,
0.0374170400486292));
#32219=CARTESIAN_POINT('Ctrl Pts',(-0.339534702539374,0.0237758430999062,
0.0425008539245673));
#32220=CARTESIAN_POINT('Ctrl Pts',(-0.329617478537296,-0.0636510452603832,
0.0460638560210726));
#32221=CARTESIAN_POINT('Ctrl Pts',(-0.315752180564557,-0.111758567679568,
0.0481010960909614));
#32222=CARTESIAN_POINT('Ctrl Pts',(-0.280687728436729,-0.19663499457563,
0.0518375549362775));
#32223=CARTESIAN_POINT('Ctrl Pts',(-0.176953832876605,-0.308707864139412,
0.0577895429568186));
#32224=CARTESIAN_POINT('Ctrl Pts',(0.0277912542949835,-0.355359243876355,
0.0659698006169508));
#32225=CARTESIAN_POINT('Ctrl Pts',(0.207256209567046,-0.285022432777545,
0.073484386523706));
#32226=CARTESIAN_POINT('Ctrl Pts',(0.31450859302708,-0.150158997366471,
0.0803284879538114));
#32227=CARTESIAN_POINT('Ctrl Pts',(0.349186611535958,0.00111014849211965,
0.0864979120385476));
#32228=CARTESIAN_POINT('Ctrl Pts',(0.314520756767304,0.152731777144028,
0.0926770234710082));
#32229=CARTESIAN_POINT('Ctrl Pts',(0.217500483746742,0.274539465175591,
0.098865768103921));
#32230=CARTESIAN_POINT('Ctrl Pts',(0.0769551264679099,0.342186713109751,
0.105064101576398));
#32231=CARTESIAN_POINT('Ctrl Pts',(-0.0793009475509065,0.342263708237282,
0.111271969453101));
#32232=CARTESIAN_POINT('Ctrl Pts',(-0.220172034550062,0.274381760656883,
0.117489309777858));
#32233=CARTESIAN_POINT('Ctrl Pts',(-0.318128621603507,0.151819046241454,
0.123716067105663));
#32234=CARTESIAN_POINT('Ctrl Pts',(-0.352617648223723,-0.000927697002303161,
0.129952164368648));
#32235=CARTESIAN_POINT('Ctrl Pts',(-0.307197248189229,-0.205991895653557,
0.138279361997572));
#32236=CARTESIAN_POINT('Ctrl Pts',(-0.0867093646975666,-0.382606488631909,
0.148711360096893));
#32237=CARTESIAN_POINT('Ctrl Pts',(0.246157896760925,-0.307226237821677,
0.16126605881999));
#32238=CARTESIAN_POINT('Ctrl Pts',(0.394548713993526,0.00121213976701099,
0.173856329664019));
#32239=CARTESIAN_POINT('Ctrl Pts',(0.270683494680064,0.25779707362797,0.184377360469391));
#32240=CARTESIAN_POINT('Ctrl Pts',(0.0784480660104459,0.348945360245205,
0.192811248605432));
#32241=CARTESIAN_POINT('Ctrl Pts',(-0.0805931042682236,0.349358375490888,
0.199145126960344));
#32242=CARTESIAN_POINT('Ctrl Pts',(-0.224524686851408,0.279914574363962,
0.205487348255157));
#32243=CARTESIAN_POINT('Ctrl Pts',(-0.324178791380424,0.155094279198964,
0.211837815149481));
#32244=CARTESIAN_POINT('Ctrl Pts',(-0.359765231562575,-0.000950160030172512,
0.218196411362682));
#32245=CARTESIAN_POINT('Ctrl Pts',(-0.324199918380757,-0.157162565812712,
0.22456305908972));
#32246=CARTESIAN_POINT('Ctrl Pts',(-0.224151419632265,-0.282543079616346,
0.230937631934188));
#32247=CARTESIAN_POINT('Ctrl Pts',(-0.0794762745603369,-0.352337612459348,
0.237319995378052));
#32248=CARTESIAN_POINT('Ctrl Pts',(0.0812906306420514,-0.352242766117238,
0.243710053380832));
#32249=CARTESIAN_POINT('Ctrl Pts',(0.242583044989387,-0.274824345329341,
0.250818566710242));
#32250=CARTESIAN_POINT('Ctrl Pts',(0.355857692111688,-0.108936398125315,
0.258648506513342));
#32251=CARTESIAN_POINT('Ctrl Pts',(0.35601905515454,0.110643209305051,0.267203260973594));
#32252=CARTESIAN_POINT('Ctrl Pts',(0.232065828412221,0.292295611594562,
0.275770669585301));
#32253=CARTESIAN_POINT('Ctrl Pts',(0.0272435837717024,0.37290401539681,
0.284350408116761));
#32254=CARTESIAN_POINT('Ctrl Pts',(-0.187879927304316,0.323810447294939,
0.292942183858905));
#32255=CARTESIAN_POINT('Ctrl Pts',(-0.325407735789747,0.17542191209667,
0.300828814614272));
#32256=CARTESIAN_POINT('Ctrl Pts',(-0.365431318619722,-0.00075089577638709,
0.308006589851792));
#32257=CARTESIAN_POINT('Ctrl Pts',(-0.329362034481868,-0.159416832712907,
0.314473213303831));
#32258=CARTESIAN_POINT('Ctrl Pts',(-0.227729428899003,-0.286678573326201,
0.320945361203317));
#32259=CARTESIAN_POINT('Ctrl Pts',(-0.0809152203341978,-0.357609127112455,
0.327424927538347));
#32260=CARTESIAN_POINT('Ctrl Pts',(0.0823028008577847,-0.357312684079966,
0.333907107762849));
#32261=CARTESIAN_POINT('Ctrl Pts',(0.229369976399687,-0.286999416296364,
0.340400245782608));
#32262=CARTESIAN_POINT('Ctrl Pts',(0.331477217034357,-0.158117971828307,
0.346888605564388));
#32263=CARTESIAN_POINT('Ctrl Pts',(0.355417803964002,-0.0537733405890617,
0.351235961881927));
#32264=CARTESIAN_POINT('Ctrl Pts',(0.355614008397637,0.000526897379297947,
0.35339086956434));
#32265=CARTESIAN_POINT('Origin',(0.33,-3.20923843055709E-16,0.369));
#32266=CARTESIAN_POINT('Origin',(0.33,-3.20923843055709E-16,0.369));
#32267=CARTESIAN_POINT('Origin',(0.33,2.0618100472869E-19,0.031));
#38592=UNCERTAINTY_MEASURE_WITH_UNIT(LENGTH_MEASURE(0.001),#38612,
'DISTANCE_ACCURACY_VALUE',
'Maximum model space distance between geometric entities at asserted c
onnectivities');
#38595=UNCERTAINTY_MEASURE_WITH_UNIT(LENGTH_MEASURE(0.001),#38612,
'DISTANCE_ACCURACY_VALUE',
'Maximum model space distance between geometric entities at asserted c
onnectivities');
#38608=(
GEOMETRIC_REPRESENTATION_CONTEXT(3)
GLOBAL_UNCERTAINTY_ASSIGNED_CONTEXT((#38592))
GLOBAL_UNIT_ASSIGNED_CONTEXT((#38612,#38614,#38615))
REPRESENTATION_CONTEXT('','3D')
);
#38611=(
GEOMETRIC_REPRESENTATION_CONTEXT(3)
GLOBAL_UNCERTAINTY_ASSIGNED_CONTEXT((#38595))
GLOBAL_UNIT_ASSIGNED_CONTEXT((#38612,#38614,#38615))
REPRESENTATION_CONTEXT('','3D')
);
#38612=(
LENGTH_UNIT()
NAMED_UNIT(*)
SI_UNIT(.CENTI.,.METRE.)
);
#38614=(
NAMED_UNIT(*)
PLANE_ANGLE_UNIT()
SI_UNIT($,.RADIAN.)
);
#38615=(
NAMED_UNIT(*)
SI_UNIT($,.STERADIAN.)
SOLID_ANGLE_UNIT()
);
#38628=SHAPE_DEFINITION_REPRESENTATION(#38643,#38679);
#38643=PRODUCT_DEFINITION_SHAPE('',$,#38695);
#38679=SHAPE_REPRESENTATION('',(#17327),#38608);
#38682=PRODUCT_DEFINITION_CONTEXT('part definition',#38729,'design');
#38695=PRODUCT_DEFINITION('2026-10-19-02-31-51-889',
'10_Preload_Compression_Spring_D7.2x0.6x4',#38710,#38682);
#38710=PRODUCT_DEFINITION_FORMATION('',$,#38743);
#38729=APPLICATION_CONTEXT(
'Core Data for Automotive Mechanical Design Process');
#38730=PRODUCT_CONTEXT('part definition',#38729,'mechanical');
#38743=PRODUCT('2026-10-19-02-31-51-889',
'10_Preload_Compression_Spring_D7.2x0.6x4',$,(#38730));
#38872=COLOUR_RGB('Grey',0.48,0.52,0.57);
#38873=FILL_AREA_STYLE_COLOUR('',#38872);
#38874=FILL_AREA_STYLE('',(#38873));
#38875=SURFACE_STYLE_FILL_AREA(#38874);
#38876=SURFACE_SIDE_STYLE('',(#38875));
#38877=SURFACE_STYLE_USAGE(.BOTH.,#38876);
#38878=PRESENTATION_STYLE_ASSIGNMENT((#38877));
ENDSEC;
END-ISO-10303-21;
